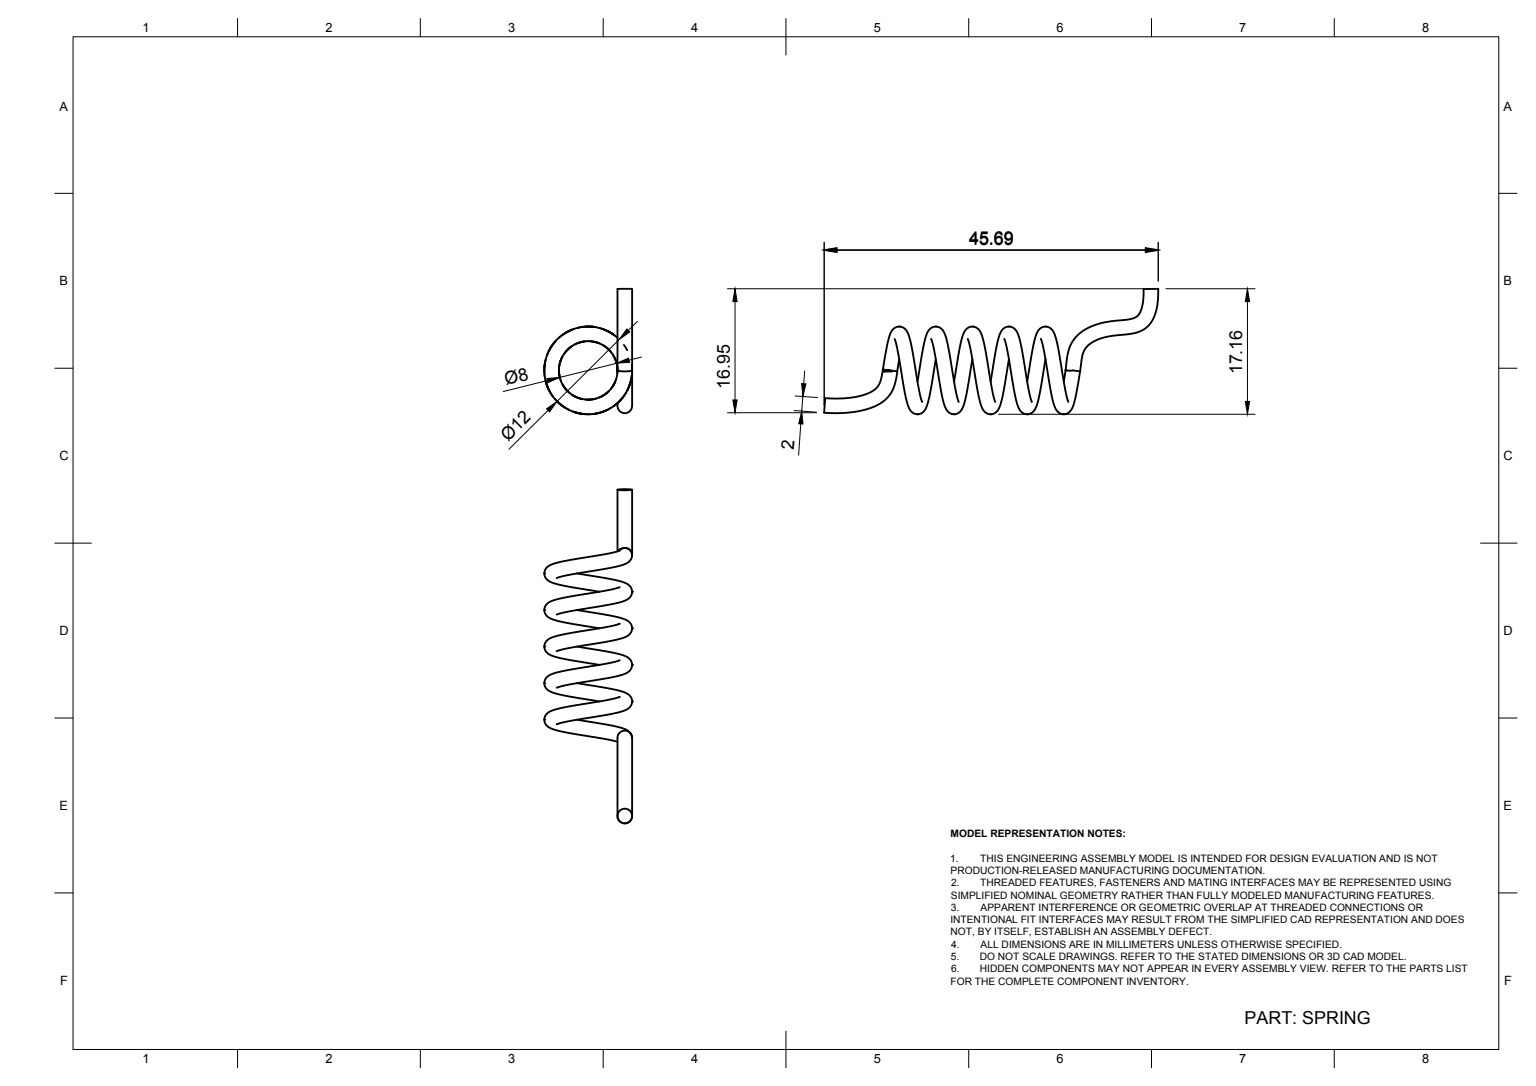
ISO-10303-21;
HEADER;
/* Generated by software containing ST-Developer
 * from STEP Tools, Inc. (www.steptools.com) 
 */

FILE_DESCRIPTION(
/* description */ (''),
/* implementation_level */ '2;1');

FILE_NAME(
/* name */ 'Spring.step',
/* time_stamp */ '2026-09-20T22:38:01+06:00',
/* author */ (''),
/* organization */ (''),
/* preprocessor_version */ 'ST-DEVELOPER v20.2',
/* originating_system */ 'Autodesk Translation Framework v15.15.0.0',
/* authorisation */ '');

FILE_SCHEMA (('AUTOMOTIVE_DESIGN { 1 0 10303 214 3 1 1 }'));
ENDSEC;

DATA;
#10=MECHANICAL_DESIGN_GEOMETRIC_PRESENTATION_REPRESENTATION('',(#86),#4079);
#43=B_SPLINE_CURVE_WITH_KNOTS('',3,(#2659,#2660,#2661,#2662,#2663,#2664,
#2665,#2666,#2667,#2668,#2669,#2670,#2671,#2672,#2673,#2674,#2675,#2676,
#2677,#2678,#2679,#2680,#2681,#2682,#2683,#2684,#2685,#2686),
 .UNSPECIFIED.,.F.,.F.,(4,3,3,3,3,3,3,3,3,4),(-0.465553767595507,-0.45230342916427,
-0.438736142747031,-0.431079433868877,-0.417558478811202,-0.404199900672923,
-0.391686604552913,-0.378322214394046,-0.374830772248012,-0.369773118077988),
 .UNSPECIFIED.);
#44=B_SPLINE_CURVE_WITH_KNOTS('',3,(#2688,#2689,#2690,#2691,#2692,#2693,
#2694,#2695,#2696,#2697),.UNSPECIFIED.,.F.,.F.,(4,2,2,2,4),(-0.09742200167385,
-0.0775242929113368,-0.0386624365460309,0.,0.00241811618144354),
 .UNSPECIFIED.);
#45=B_SPLINE_CURVE_WITH_KNOTS('',3,(#2702,#2703,#2704,#2705,#2706,#2707,
#2708,#2709,#2710,#2711),.UNSPECIFIED.,.F.,.F.,(4,3,3,4),(-0.657219142658169,
-0.648664678619421,-0.598426048115365,-0.569492481999336),.UNSPECIFIED.);
#46=B_SPLINE_CURVE_WITH_KNOTS('',3,(#2712,#2713,#2714,#2715,#2716,#2717,
#2718,#2719,#2720,#2721),.UNSPECIFIED.,.F.,.F.,(4,3,3,4),(-0.489269526390867,
-0.47602824474659,-0.470821216724862,-0.465553767595507),.UNSPECIFIED.);
#47=B_SPLINE_CURVE_WITH_KNOTS('',3,(#2723,#2724,#2725,#2726,#2727,#2728,
#2729,#2730,#2731),.UNSPECIFIED.,.F.,.F.,(4,1,1,1,1,1,4),(0.0132171477861262,
0.142857142857143,0.285714285714286,0.428571428571429,0.571428571428571,
0.857142857142857,1.),.UNSPECIFIED.);
#48=B_SPLINE_CURVE_WITH_KNOTS('',3,(#3403,#3404,#3405,#3406,#3407,#3408,
#3409,#3410,#3411,#3412,#3413,#3414,#3415,#3416,#3417,#3418,#3419,#3420,
#3421,#3422,#3423,#3424,#3425),.UNSPECIFIED.,.F.,.F.,(4,2,3,2,2,2,2,2,2,
2,4),(0.587267836178956,0.604560146171109,0.626248329271999,0.664698946888708,
0.70347541138122,0.74264809527987,0.78210152700143,0.821492769940296,0.860375715352057,
0.898588405045022,0.900352617840992),.UNSPECIFIED.);
#49=B_SPLINE_CURVE_WITH_KNOTS('',3,(#3427,#3428,#3429,#3430,#3431,#3432,
#3433,#3434,#3435,#3436,#3437,#3438,#3439,#3440,#3441,#3442,#3443,#3444,
#3445,#3446,#3447,#3448,#3449,#3450,#3451,#3452,#3453,#3454,#3455,#3456,
#3457,#3458,#3459,#3460,#3461,#3462,#3463,#3464,#3465,#3466,#3467,#3468,
#3469,#3470,#3471,#3472,#3473,#3474,#3475,#3476,#3477,#3478,#3479,#3480,
#3481,#3482,#3483,#3484,#3485,#3486,#3487,#3488,#3489,#3490,#3491,#3492,
#3493),.UNSPECIFIED.,.F.,.F.,(4,1,1,1,1,1,1,1,1,1,1,1,1,1,1,1,1,1,1,1,1,
1,1,1,1,1,1,1,1,1,1,1,1,1,1,1,1,1,1,1,1,1,1,1,1,1,1,1,1,1,1,1,1,1,1,1,1,
1,1,1,1,1,1,1,4),(0.,0.464577110944849,0.95586837165839,1.44715963237193,
1.93845089308547,2.42974215379901,2.92103341451255,3.41232467522609,3.90361593593964,
4.39490719665318,4.88619845736672,5.37748971808026,5.8687809787938,6.36007223950734,
6.85136350022088,7.34265476093442,7.83394602164796,8.3252372823615,8.81652854307505,
9.30781980378859,9.79911106450213,10.2904023252157,10.7816935859292,11.2729848466427,
11.7642761073563,12.2555673680698,12.7468586287834,13.2381498894969,13.7294411502105,
14.220732410924,14.7120236716375,15.2033149323511,15.6946061930646,16.1858974537782,
16.6771887144917,17.1684799752052,17.6597712359188,18.1510624966323,18.6423537573459,
19.1336450180594,19.6249362787729,20.1162275394865,20.6075188002,21.0988100609136,
21.5901013216271,22.0813925823407,22.5726838430542,23.0639751037677,23.5552663644813,
24.0465576251948,24.5378488859084,25.0291401466219,25.5204314073354,26.011722668049,
26.5030139287625,26.9943051894761,27.4855964501896,27.9768877109031,28.4681789716167,
28.9594702323302,29.4507614930438,29.9420527537573,30.4333440144708,30.9246352751844,
31.4159265358979),.UNSPECIFIED.);
#50=B_SPLINE_CURVE_WITH_KNOTS('',3,(#3495,#3496,#3497,#3498,#3499,#3500,
#3501,#3502,#3503,#3504,#3505,#3506,#3507,#3508,#3509,#3510,#3511,#3512,
#3513,#3514),.UNSPECIFIED.,.F.,.F.,(4,2,2,2,2,2,2,2,2,4),(-0.313052705156199,
-0.292609441796844,-0.272153993775093,-0.233472325120928,-0.194370984993977,
-0.154905297587714,-0.115391052867927,-0.0763129985395409,-0.0379453287021336,
0.),.UNSPECIFIED.);
#51=B_SPLINE_CURVE_WITH_KNOTS('',3,(#3516,#3517,#3518,#3519,#3520,#3521,
#3522,#3523,#3524,#3525,#3526,#3527,#3528,#3529,#3530,#3531),
 .UNSPECIFIED.,.F.,.F.,(4,3,3,3,3,4),(-0.0024248849541149,0.,0.0138283319525736,
0.0273768962823761,0.0362935842092716,0.0434201122759664),.UNSPECIFIED.);
#52=B_SPLINE_CURVE_WITH_KNOTS('',3,(#3533,#3534,#3535,#3536,#3537,#3538),
 .UNSPECIFIED.,.F.,.F.,(4,2,4),(-0.0515505060017679,-0.0391387739403107,
0.),.UNSPECIFIED.);
#53=B_SPLINE_CURVE_WITH_KNOTS('',3,(#3542,#3543,#3544,#3545,#3546,#3547,
#3548,#3549,#3550,#3551,#3552,#3553,#3554,#3555,#3556,#3557,#3558,#3559,
#3560,#3561),.UNSPECIFIED.,.F.,.F.,(4,2,2,2,2,2,2,2,2,4),(-0.313052705156207,
-0.29260944179685,-0.272153993775096,-0.233472325120924,-0.194370984993967,
-0.154905297587702,-0.11539105286792,-0.0763129985395404,-0.0379453287021338,
0.),.UNSPECIFIED.);
#54=B_SPLINE_CURVE_WITH_KNOTS('',3,(#3563,#3564,#3565,#3566,#3567,#3568,
#3569,#3570,#3571,#3572,#3573,#3574,#3575,#3576,#3577,#3578,#3579,#3580,
#3581,#3582,#3583,#3584,#3585,#3586,#3587,#3588,#3589,#3590,#3591,#3592,
#3593,#3594,#3595,#3596),.UNSPECIFIED.,.F.,.F.,(4,3,3,3,3,3,3,3,3,3,3,4),
(0.377352254196932,0.390588465654341,0.403867575958707,0.41718187397498,
0.429352359462404,0.437218808334642,0.450427222970435,0.463782588613302,
0.468146972739535,0.481501401691605,0.494833441685106,0.497267224677679),
 .UNSPECIFIED.);
#55=B_SPLINE_CURVE_WITH_KNOTS('',3,(#3600,#3601,#3602,#3603,#3604,#3605,
#3606,#3607,#3608,#3609,#3610,#3611,#3612,#3613,#3614,#3615,#3616,#3617,
#3618,#3619,#3620,#3621,#3622,#3623,#3624,#3625,#3626,#3627),
 .UNSPECIFIED.,.F.,.F.,(4,3,3,3,3,3,3,3,3,4),(0.458621120799817,0.464048968999107,
0.469643578756217,0.482746851650584,0.496256676637028,0.508878670584022,
0.522421915099756,0.535791652499991,0.548459753273671,0.554671659389392),
 .UNSPECIFIED.);
#56=B_SPLINE_CURVE_WITH_KNOTS('',3,(#3888,#3889,#3890,#3891,#3892,#3893,
#3894,#3895,#3896,#3897),.UNSPECIFIED.,.F.,.F.,(4,3,3,4),(-0.319964114535563,
-0.319531325306217,-0.229500308639694,-0.144878157103041),.UNSPECIFIED.);
#57=B_SPLINE_CURVE_WITH_KNOTS('',3,(#3900,#3901,#3902,#3903,#3904,#3905,
#3906,#3907,#3908,#3909,#3910,#3911,#3912,#3913,#3914,#3915,#3916,#3917,
#3918,#3919,#3920,#3921,#3922,#3923),.UNSPECIFIED.,.F.,.F.,(4,1,1,1,1,1,
1,1,1,1,1,1,1,1,1,1,1,1,1,1,1,4),(0.,0.025,0.05,0.1,0.15,0.175,0.2,0.3,
0.4,0.425,0.45,0.5,0.55,0.575,0.6,0.7,0.75,0.8,0.825,0.85,0.9,1.),
 .UNSPECIFIED.);
#58=B_SPLINE_SURFACE_WITH_KNOTS('',3,3,((#2567,#2568,#2569,#2570,#2571,
#2572,#2573,#2574,#2575),(#2576,#2577,#2578,#2579,#2580,#2581,#2582,#2583,
#2584),(#2585,#2586,#2587,#2588,#2589,#2590,#2591,#2592,#2593),(#2594,#2595,
#2596,#2597,#2598,#2599,#2600,#2601,#2602),(#2603,#2604,#2605,#2606,#2607,
#2608,#2609,#2610,#2611),(#2612,#2613,#2614,#2615,#2616,#2617,#2618,#2619,
#2620),(#2621,#2622,#2623,#2624,#2625,#2626,#2627,#2628,#2629),(#2630,#2631,
#2632,#2633,#2634,#2635,#2636,#2637,#2638),(#2639,#2640,#2641,#2642,#2643,
#2644,#2645,#2646,#2647),(#2648,#2649,#2650,#2651,#2652,#2653,#2654,#2655,
#2656)),.UNSPECIFIED.,.T.,.F.,.F.,(4,1,1,1,1,1,1,4),(4,1,1,1,1,1,4),(-3.14159265359034,
-2.2439947525646,-1.34639685153886,-0.448798950513122,0.448798950512615,
1.34639685153835,2.24399475256409,3.14159265358983),(0.,0.142857142857143,
0.285714285714286,0.428571428571429,0.571428571428571,0.857142857142857,
1.),.UNSPECIFIED.);
#59=B_SPLINE_SURFACE_WITH_KNOTS('',3,3,((#2733,#2734,#2735,#2736,#2737,
#2738,#2739,#2740,#2741,#2742,#2743,#2744,#2745,#2746,#2747,#2748,#2749,
#2750,#2751,#2752,#2753,#2754,#2755,#2756,#2757,#2758,#2759,#2760,#2761,
#2762,#2763,#2764,#2765,#2766,#2767,#2768,#2769,#2770,#2771,#2772,#2773,
#2774,#2775,#2776,#2777,#2778,#2779,#2780,#2781,#2782,#2783,#2784,#2785,
#2786,#2787,#2788,#2789,#2790,#2791,#2792,#2793,#2794,#2795,#2796,#2797,
#2798,#2799),(#2800,#2801,#2802,#2803,#2804,#2805,#2806,#2807,#2808,#2809,
#2810,#2811,#2812,#2813,#2814,#2815,#2816,#2817,#2818,#2819,#2820,#2821,
#2822,#2823,#2824,#2825,#2826,#2827,#2828,#2829,#2830,#2831,#2832,#2833,
#2834,#2835,#2836,#2837,#2838,#2839,#2840,#2841,#2842,#2843,#2844,#2845,
#2846,#2847,#2848,#2849,#2850,#2851,#2852,#2853,#2854,#2855,#2856,#2857,
#2858,#2859,#2860,#2861,#2862,#2863,#2864,#2865,#2866),(#2867,#2868,#2869,
#2870,#2871,#2872,#2873,#2874,#2875,#2876,#2877,#2878,#2879,#2880,#2881,
#2882,#2883,#2884,#2885,#2886,#2887,#2888,#2889,#2890,#2891,#2892,#2893,
#2894,#2895,#2896,#2897,#2898,#2899,#2900,#2901,#2902,#2903,#2904,#2905,
#2906,#2907,#2908,#2909,#2910,#2911,#2912,#2913,#2914,#2915,#2916,#2917,
#2918,#2919,#2920,#2921,#2922,#2923,#2924,#2925,#2926,#2927,#2928,#2929,
#2930,#2931,#2932,#2933),(#2934,#2935,#2936,#2937,#2938,#2939,#2940,#2941,
#2942,#2943,#2944,#2945,#2946,#2947,#2948,#2949,#2950,#2951,#2952,#2953,
#2954,#2955,#2956,#2957,#2958,#2959,#2960,#2961,#2962,#2963,#2964,#2965,
#2966,#2967,#2968,#2969,#2970,#2971,#2972,#2973,#2974,#2975,#2976,#2977,
#2978,#2979,#2980,#2981,#2982,#2983,#2984,#2985,#2986,#2987,#2988,#2989,
#2990,#2991,#2992,#2993,#2994,#2995,#2996,#2997,#2998,#2999,#3000),(#3001,
#3002,#3003,#3004,#3005,#3006,#3007,#3008,#3009,#3010,#3011,#3012,#3013,
#3014,#3015,#3016,#3017,#3018,#3019,#3020,#3021,#3022,#3023,#3024,#3025,
#3026,#3027,#3028,#3029,#3030,#3031,#3032,#3033,#3034,#3035,#3036,#3037,
#3038,#3039,#3040,#3041,#3042,#3043,#3044,#3045,#3046,#3047,#3048,#3049,
#3050,#3051,#3052,#3053,#3054,#3055,#3056,#3057,#3058,#3059,#3060,#3061,
#3062,#3063,#3064,#3065,#3066,#3067),(#3068,#3069,#3070,#3071,#3072,#3073,
#3074,#3075,#3076,#3077,#3078,#3079,#3080,#3081,#3082,#3083,#3084,#3085,
#3086,#3087,#3088,#3089,#3090,#3091,#3092,#3093,#3094,#3095,#3096,#3097,
#3098,#3099,#3100,#3101,#3102,#3103,#3104,#3105,#3106,#3107,#3108,#3109,
#3110,#3111,#3112,#3113,#3114,#3115,#3116,#3117,#3118,#3119,#3120,#3121,
#3122,#3123,#3124,#3125,#3126,#3127,#3128,#3129,#3130,#3131,#3132,#3133,
#3134),(#3135,#3136,#3137,#3138,#3139,#3140,#3141,#3142,#3143,#3144,#3145,
#3146,#3147,#3148,#3149,#3150,#3151,#3152,#3153,#3154,#3155,#3156,#3157,
#3158,#3159,#3160,#3161,#3162,#3163,#3164,#3165,#3166,#3167,#3168,#3169,
#3170,#3171,#3172,#3173,#3174,#3175,#3176,#3177,#3178,#3179,#3180,#3181,
#3182,#3183,#3184,#3185,#3186,#3187,#3188,#3189,#3190,#3191,#3192,#3193,
#3194,#3195,#3196,#3197,#3198,#3199,#3200,#3201),(#3202,#3203,#3204,#3205,
#3206,#3207,#3208,#3209,#3210,#3211,#3212,#3213,#3214,#3215,#3216,#3217,
#3218,#3219,#3220,#3221,#3222,#3223,#3224,#3225,#3226,#3227,#3228,#3229,
#3230,#3231,#3232,#3233,#3234,#3235,#3236,#3237,#3238,#3239,#3240,#3241,
#3242,#3243,#3244,#3245,#3246,#3247,#3248,#3249,#3250,#3251,#3252,#3253,
#3254,#3255,#3256,#3257,#3258,#3259,#3260,#3261,#3262,#3263,#3264,#3265,
#3266,#3267,#3268),(#3269,#3270,#3271,#3272,#3273,#3274,#3275,#3276,#3277,
#3278,#3279,#3280,#3281,#3282,#3283,#3284,#3285,#3286,#3287,#3288,#3289,
#3290,#3291,#3292,#3293,#3294,#3295,#3296,#3297,#3298,#3299,#3300,#3301,
#3302,#3303,#3304,#3305,#3306,#3307,#3308,#3309,#3310,#3311,#3312,#3313,
#3314,#3315,#3316,#3317,#3318,#3319,#3320,#3321,#3322,#3323,#3324,#3325,
#3326,#3327,#3328,#3329,#3330,#3331,#3332,#3333,#3334,#3335),(#3336,#3337,
#3338,#3339,#3340,#3341,#3342,#3343,#3344,#3345,#3346,#3347,#3348,#3349,
#3350,#3351,#3352,#3353,#3354,#3355,#3356,#3357,#3358,#3359,#3360,#3361,
#3362,#3363,#3364,#3365,#3366,#3367,#3368,#3369,#3370,#3371,#3372,#3373,
#3374,#3375,#3376,#3377,#3378,#3379,#3380,#3381,#3382,#3383,#3384,#3385,
#3386,#3387,#3388,#3389,#3390,#3391,#3392,#3393,#3394,#3395,#3396,#3397,
#3398,#3399,#3400,#3401,#3402)),.UNSPECIFIED.,.T.,.F.,.F.,(4,1,1,1,1,1,
1,4),(4,1,1,1,1,1,1,1,1,1,1,1,1,1,1,1,1,1,1,1,1,1,1,1,1,1,1,1,1,1,1,1,1,
1,1,1,1,1,1,1,1,1,1,1,1,1,1,1,1,1,1,1,1,1,1,1,1,1,1,1,1,1,1,1,4),(-3.14159265358979,
-2.24399475256414,-1.34639685153848,-0.448798950512828,0.448798950512828,
1.34639685153848,2.24399475256414,3.14159265358979),(-0.0267141497686917,
0.464577110944849,0.95586837165839,1.44715963237193,1.93845089308547,2.42974215379901,
2.92103341451255,3.41232467522609,3.90361593593964,4.39490719665318,4.88619845736672,
5.37748971808026,5.8687809787938,6.36007223950734,6.85136350022088,7.34265476093442,
7.83394602164796,8.3252372823615,8.81652854307505,9.30781980378859,9.79911106450213,
10.2904023252157,10.7816935859292,11.2729848466427,11.7642761073563,12.2555673680698,
12.7468586287834,13.2381498894969,13.7294411502105,14.220732410924,14.7120236716375,
15.2033149323511,15.6946061930646,16.1858974537782,16.6771887144917,17.1684799752052,
17.6597712359188,18.1510624966323,18.6423537573459,19.1336450180594,19.6249362787729,
20.1162275394865,20.6075188002,21.0988100609136,21.5901013216271,22.0813925823407,
22.5726838430542,23.0639751037677,23.5552663644813,24.0465576251948,24.5378488859084,
25.0291401466219,25.5204314073354,26.011722668049,26.5030139287625,26.9943051894761,
27.4855964501896,27.9768877109031,28.4681789716167,28.9594702323302,29.4507614930438,
29.9420527537573,30.4333440144708,30.9246352751844,31.4159265358979),
 .UNSPECIFIED.);
#60=B_SPLINE_SURFACE_WITH_KNOTS('',3,3,((#3628,#3629,#3630,#3631,#3632,
#3633,#3634,#3635,#3636,#3637,#3638,#3639,#3640,#3641,#3642,#3643,#3644,
#3645,#3646,#3647,#3648,#3649,#3650,#3651,#3652,#3653),(#3654,#3655,#3656,
#3657,#3658,#3659,#3660,#3661,#3662,#3663,#3664,#3665,#3666,#3667,#3668,
#3669,#3670,#3671,#3672,#3673,#3674,#3675,#3676,#3677,#3678,#3679),(#3680,
#3681,#3682,#3683,#3684,#3685,#3686,#3687,#3688,#3689,#3690,#3691,#3692,
#3693,#3694,#3695,#3696,#3697,#3698,#3699,#3700,#3701,#3702,#3703,#3704,
#3705),(#3706,#3707,#3708,#3709,#3710,#3711,#3712,#3713,#3714,#3715,#3716,
#3717,#3718,#3719,#3720,#3721,#3722,#3723,#3724,#3725,#3726,#3727,#3728,
#3729,#3730,#3731),(#3732,#3733,#3734,#3735,#3736,#3737,#3738,#3739,#3740,
#3741,#3742,#3743,#3744,#3745,#3746,#3747,#3748,#3749,#3750,#3751,#3752,
#3753,#3754,#3755,#3756,#3757),(#3758,#3759,#3760,#3761,#3762,#3763,#3764,
#3765,#3766,#3767,#3768,#3769,#3770,#3771,#3772,#3773,#3774,#3775,#3776,
#3777,#3778,#3779,#3780,#3781,#3782,#3783),(#3784,#3785,#3786,#3787,#3788,
#3789,#3790,#3791,#3792,#3793,#3794,#3795,#3796,#3797,#3798,#3799,#3800,
#3801,#3802,#3803,#3804,#3805,#3806,#3807,#3808,#3809),(#3810,#3811,#3812,
#3813,#3814,#3815,#3816,#3817,#3818,#3819,#3820,#3821,#3822,#3823,#3824,
#3825,#3826,#3827,#3828,#3829,#3830,#3831,#3832,#3833,#3834,#3835),(#3836,
#3837,#3838,#3839,#3840,#3841,#3842,#3843,#3844,#3845,#3846,#3847,#3848,
#3849,#3850,#3851,#3852,#3853,#3854,#3855,#3856,#3857,#3858,#3859,#3860,
#3861),(#3862,#3863,#3864,#3865,#3866,#3867,#3868,#3869,#3870,#3871,#3872,
#3873,#3874,#3875,#3876,#3877,#3878,#3879,#3880,#3881,#3882,#3883,#3884,
#3885,#3886,#3887)),.UNSPECIFIED.,.T.,.F.,.F.,(4,1,1,1,1,1,1,4),(4,2,1,
1,1,1,1,1,1,1,1,1,1,1,1,1,1,1,1,1,1,1,4),(-3.14159265358979,-2.24399475256414,
-1.34639685153848,-0.448798950512828,0.448798950512828,1.34639685153848,
2.24399475256414,3.14159265358979),(-0.00680747846147418,0.,0.025,0.05,
0.1,0.15,0.175,0.2,0.3,0.4,0.425,0.45,0.5,0.55,0.575,0.6,0.7,0.75,0.8,0.825,
0.85,0.9,1.),.UNSPECIFIED.);
#61=B_SPLINE_SURFACE_WITH_KNOTS('',3,3,((#3925,#3926,#3927,#3928),(#3929,
#3930,#3931,#3932),(#3933,#3934,#3935,#3936),(#3937,#3938,#3939,#3940),
(#3941,#3942,#3943,#3944)),.UNSPECIFIED.,.F.,.F.,.F.,(4,1,4),(4,4),(-0.950877784735382,
-0.352362581588169,0.246152621559044),(-0.0375396701634702,0.),
 .UNSPECIFIED.);
#70=SHAPE_REPRESENTATION_RELATIONSHIP('SRR','None',#4113,#78);
#78=ADVANCED_BREP_SHAPE_REPRESENTATION('',(#94),#4073);
#86=STYLED_ITEM('',(#4162),#94);
#94=MANIFOLD_SOLID_BREP('Spring',#1445);
#150=CIRCLE('',#1633,1.);
#151=CIRCLE('',#1634,1.);
#152=CIRCLE('',#1635,1.);
#153=CIRCLE('',#1636,1.);
#154=CIRCLE('',#1637,1.);
#155=CIRCLE('',#1640,1.);
#156=CIRCLE('',#1641,1.);
#244=FACE_OUTER_BOUND('',#332,.T.);
#245=FACE_OUTER_BOUND('',#333,.T.);
#246=FACE_OUTER_BOUND('',#334,.T.);
#247=FACE_OUTER_BOUND('',#335,.T.);
#248=FACE_OUTER_BOUND('',#336,.T.);
#249=FACE_OUTER_BOUND('',#337,.T.);
#250=FACE_OUTER_BOUND('',#338,.T.);
#251=FACE_OUTER_BOUND('',#339,.T.);
#252=FACE_OUTER_BOUND('',#340,.T.);
#253=FACE_OUTER_BOUND('',#341,.T.);
#254=FACE_OUTER_BOUND('',#342,.T.);
#255=FACE_OUTER_BOUND('',#343,.T.);
#256=FACE_OUTER_BOUND('',#344,.T.);
#332=EDGE_LOOP('',(#1177,#1178,#1179,#1180,#1181,#1182,#1183,#1184,#1185));
#333=EDGE_LOOP('',(#1186,#1187,#1188,#1189,#1190,#1191,#1192,#1193,#1194));
#334=EDGE_LOOP('',(#1195,#1196,#1197));
#335=EDGE_LOOP('',(#1198,#1199,#1200));
#336=EDGE_LOOP('',(#1201,#1202,#1203,#1204,#1205,#1206,#1207));
#337=EDGE_LOOP('',(#1208,#1209,#1210));
#338=EDGE_LOOP('',(#1211,#1212));
#339=EDGE_LOOP('',(#1213,#1214));
#340=EDGE_LOOP('',(#1215));
#341=EDGE_LOOP('',(#1216,#1217,#1218,#1219));
#342=EDGE_LOOP('',(#1220,#1221));
#343=EDGE_LOOP('',(#1222));
#344=EDGE_LOOP('',(#1223,#1224));
#452=LINE('',#3599,#565);
#453=LINE('',#3949,#566);
#565=VECTOR('',#1979,10.);
#566=VECTOR('',#1992,10.);
#683=VERTEX_POINT('',#2657);
#684=VERTEX_POINT('',#2658);
#685=VERTEX_POINT('',#2687);
#686=VERTEX_POINT('',#2698);
#687=VERTEX_POINT('',#2701);
#688=VERTEX_POINT('',#2722);
#689=VERTEX_POINT('',#3426);
#690=VERTEX_POINT('',#3494);
#691=VERTEX_POINT('',#3515);
#692=VERTEX_POINT('',#3532);
#693=VERTEX_POINT('',#3539);
#694=VERTEX_POINT('',#3598);
#695=VERTEX_POINT('',#3899);
#853=EDGE_CURVE('',#683,#684,#43,.T.);
#854=EDGE_CURVE('',#684,#685,#44,.T.);
#855=EDGE_CURVE('',#685,#686,#150,.T.);
#856=EDGE_CURVE('',#686,#685,#151,.T.);
#857=EDGE_CURVE('',#685,#687,#45,.T.);
#858=EDGE_CURVE('',#687,#683,#46,.T.);
#859=EDGE_CURVE('',#683,#688,#47,.T.);
#860=EDGE_CURVE('',#688,#688,#152,.T.);
#861=EDGE_CURVE('',#686,#685,#48,.T.);
#862=EDGE_CURVE('',#686,#689,#49,.T.);
#863=EDGE_CURVE('',#689,#690,#50,.T.);
#864=EDGE_CURVE('',#690,#691,#51,.T.);
#865=EDGE_CURVE('',#691,#692,#52,.T.);
#866=EDGE_CURVE('',#693,#692,#153,.T.);
#867=EDGE_CURVE('',#693,#689,#154,.T.);
#868=EDGE_CURVE('',#686,#685,#53,.T.);
#869=EDGE_CURVE('',#684,#687,#54,.T.);
#870=EDGE_CURVE('',#693,#694,#452,.T.);
#871=EDGE_CURVE('',#694,#689,#55,.T.);
#872=EDGE_CURVE('',#691,#694,#56,.T.);
#873=EDGE_CURVE('',#690,#689,#155,.T.);
#874=EDGE_CURVE('',#689,#695,#57,.T.);
#875=EDGE_CURVE('',#695,#695,#156,.T.);
#876=EDGE_CURVE('',#692,#693,#453,.F.);
#1177=ORIENTED_EDGE('',*,*,#853,.T.);
#1178=ORIENTED_EDGE('',*,*,#854,.T.);
#1179=ORIENTED_EDGE('',*,*,#855,.T.);
#1180=ORIENTED_EDGE('',*,*,#856,.T.);
#1181=ORIENTED_EDGE('',*,*,#857,.T.);
#1182=ORIENTED_EDGE('',*,*,#858,.T.);
#1183=ORIENTED_EDGE('',*,*,#859,.T.);
#1184=ORIENTED_EDGE('',*,*,#860,.F.);
#1185=ORIENTED_EDGE('',*,*,#859,.F.);
#1186=ORIENTED_EDGE('',*,*,#861,.F.);
#1187=ORIENTED_EDGE('',*,*,#862,.T.);
#1188=ORIENTED_EDGE('',*,*,#863,.T.);
#1189=ORIENTED_EDGE('',*,*,#864,.T.);
#1190=ORIENTED_EDGE('',*,*,#865,.T.);
#1191=ORIENTED_EDGE('',*,*,#866,.F.);
#1192=ORIENTED_EDGE('',*,*,#867,.T.);
#1193=ORIENTED_EDGE('',*,*,#862,.F.);
#1194=ORIENTED_EDGE('',*,*,#868,.T.);
#1195=ORIENTED_EDGE('',*,*,#858,.F.);
#1196=ORIENTED_EDGE('',*,*,#869,.F.);
#1197=ORIENTED_EDGE('',*,*,#853,.F.);
#1198=ORIENTED_EDGE('',*,*,#867,.F.);
#1199=ORIENTED_EDGE('',*,*,#870,.T.);
#1200=ORIENTED_EDGE('',*,*,#871,.T.);
#1201=ORIENTED_EDGE('',*,*,#872,.F.);
#1202=ORIENTED_EDGE('',*,*,#864,.F.);
#1203=ORIENTED_EDGE('',*,*,#873,.T.);
#1204=ORIENTED_EDGE('',*,*,#874,.T.);
#1205=ORIENTED_EDGE('',*,*,#875,.F.);
#1206=ORIENTED_EDGE('',*,*,#874,.F.);
#1207=ORIENTED_EDGE('',*,*,#871,.F.);
#1208=ORIENTED_EDGE('',*,*,#854,.F.);
#1209=ORIENTED_EDGE('',*,*,#869,.T.);
#1210=ORIENTED_EDGE('',*,*,#857,.F.);
#1211=ORIENTED_EDGE('',*,*,#855,.F.);
#1212=ORIENTED_EDGE('',*,*,#868,.F.);
#1213=ORIENTED_EDGE('',*,*,#861,.T.);
#1214=ORIENTED_EDGE('',*,*,#856,.F.);
#1215=ORIENTED_EDGE('',*,*,#860,.T.);
#1216=ORIENTED_EDGE('',*,*,#865,.F.);
#1217=ORIENTED_EDGE('',*,*,#872,.T.);
#1218=ORIENTED_EDGE('',*,*,#870,.F.);
#1219=ORIENTED_EDGE('',*,*,#876,.F.);
#1220=ORIENTED_EDGE('',*,*,#863,.F.);
#1221=ORIENTED_EDGE('',*,*,#873,.F.);
#1222=ORIENTED_EDGE('',*,*,#875,.T.);
#1223=ORIENTED_EDGE('',*,*,#876,.T.);
#1224=ORIENTED_EDGE('',*,*,#866,.T.);
#1332=PLANE('',#1638);
#1333=PLANE('',#1639);
#1334=PLANE('',#1642);
#1335=PLANE('',#1643);
#1336=PLANE('',#1644);
#1337=PLANE('',#1645);
#1338=PLANE('',#1646);
#1339=PLANE('',#1647);
#1340=PLANE('',#1648);
#1406=ADVANCED_FACE('',(#244),#58,.T.);
#1407=ADVANCED_FACE('',(#245),#59,.T.);
#1408=ADVANCED_FACE('',(#246),#1332,.F.);
#1409=ADVANCED_FACE('',(#247),#1333,.F.);
#1410=ADVANCED_FACE('',(#248),#60,.T.);
#1411=ADVANCED_FACE('',(#249),#61,.T.);
#1412=ADVANCED_FACE('',(#250),#1334,.F.);
#1413=ADVANCED_FACE('',(#251),#1335,.F.);
#1414=ADVANCED_FACE('',(#252),#1336,.T.);
#1415=ADVANCED_FACE('',(#253),#1337,.F.);
#1416=ADVANCED_FACE('',(#254),#1338,.F.);
#1417=ADVANCED_FACE('',(#255),#1339,.T.);
#1418=ADVANCED_FACE('',(#256),#1340,.T.);
#1445=CLOSED_SHELL('',(#1406,#1407,#1408,#1409,#1410,#1411,#1412,#1413,
#1414,#1415,#1416,#1417,#1418));
#1632=AXIS2_PLACEMENT_3D('',#2566,#1963,#1964);
#1633=AXIS2_PLACEMENT_3D('',#2699,#1965,#1966);
#1634=AXIS2_PLACEMENT_3D('',#2700,#1967,#1968);
#1635=AXIS2_PLACEMENT_3D('',#2732,#1969,#1970);
#1636=AXIS2_PLACEMENT_3D('',#3540,#1971,#1972);
#1637=AXIS2_PLACEMENT_3D('',#3541,#1973,#1974);
#1638=AXIS2_PLACEMENT_3D('',#3562,#1975,#1976);
#1639=AXIS2_PLACEMENT_3D('',#3597,#1977,#1978);
#1640=AXIS2_PLACEMENT_3D('',#3898,#1980,#1981);
#1641=AXIS2_PLACEMENT_3D('',#3924,#1982,#1983);
#1642=AXIS2_PLACEMENT_3D('',#3945,#1984,#1985);
#1643=AXIS2_PLACEMENT_3D('',#3946,#1986,#1987);
#1644=AXIS2_PLACEMENT_3D('',#3947,#1988,#1989);
#1645=AXIS2_PLACEMENT_3D('',#3948,#1990,#1991);
#1646=AXIS2_PLACEMENT_3D('',#3950,#1993,#1994);
#1647=AXIS2_PLACEMENT_3D('',#3951,#1995,#1996);
#1648=AXIS2_PLACEMENT_3D('',#3952,#1997,#1998);
#1963=DIRECTION('axis',(0.,0.,1.));
#1964=DIRECTION('refdir',(1.,0.,0.));
#1965=DIRECTION('center_axis',(0.,-0.991319117631768,-0.131477781460493));
#1966=DIRECTION('ref_axis',(1.,0.,0.));
#1967=DIRECTION('center_axis',(0.,-0.991319117631768,-0.131477781460493));
#1968=DIRECTION('ref_axis',(1.,0.,0.));
#1969=DIRECTION('center_axis',(0.,0.072334353589932,-0.997380439597011));
#1970=DIRECTION('ref_axis',(1.,0.,0.));
#1971=DIRECTION('center_axis',(1.22464679914735E-15,1.,0.));
#1972=DIRECTION('ref_axis',(-1.,1.22464679914735E-15,0.));
#1973=DIRECTION('center_axis',(-1.22464679914735E-15,-1.,0.));
#1974=DIRECTION('ref_axis',(-1.,1.22464679914735E-15,0.));
#1975=DIRECTION('center_axis',(0.,1.,0.));
#1976=DIRECTION('ref_axis',(0.,0.,1.));
#1977=DIRECTION('center_axis',(1.22464679914735E-15,1.,0.));
#1978=DIRECTION('ref_axis',(0.,0.,1.));
#1979=DIRECTION('',(1.,-1.22464679914735E-15,9.23361932986486E-15));
#1980=DIRECTION('center_axis',(0.,0.991319117631768,0.13147778146049));
#1981=DIRECTION('ref_axis',(-1.,0.,0.));
#1982=DIRECTION('center_axis',(0.,0.999879786123581,-0.0155052668942604));
#1983=DIRECTION('ref_axis',(-1.,0.,0.));
#1984=DIRECTION('center_axis',(0.,-0.991319117631768,-0.131477781460493));
#1985=DIRECTION('ref_axis',(0.,0.131477781460493,-0.991319117631768));
#1986=DIRECTION('center_axis',(0.,-0.991319117631768,-0.131477781460493));
#1987=DIRECTION('ref_axis',(0.,0.131477781460493,-0.991319117631768));
#1988=DIRECTION('center_axis',(0.,0.072334353589932,-0.997380439597011));
#1989=DIRECTION('ref_axis',(0.,0.997380439597011,0.072334353589932));
#1990=DIRECTION('center_axis',(0.,0.991319117631768,0.13147778146049));
#1991=DIRECTION('ref_axis',(0.,-0.13147778146049,0.991319117631768));
#1992=DIRECTION('',(-1.,1.22464679914735E-15,-9.23361932986486E-15));
#1993=DIRECTION('center_axis',(0.,0.991319117631768,0.13147778146049));
#1994=DIRECTION('ref_axis',(0.,-0.13147778146049,0.991319117631768));
#1995=DIRECTION('center_axis',(0.,0.999879786123581,-0.0155052668942604));
#1996=DIRECTION('ref_axis',(0.,0.0155052668942604,0.999879786123581));
#1997=DIRECTION('center_axis',(1.22464679914735E-15,1.,0.));
#1998=DIRECTION('ref_axis',(0.,0.,1.));
#2566=CARTESIAN_POINT('',(0.,0.,0.));
#2567=CARTESIAN_POINT('Ctrl Pts',(56.6181736442213,-16.9999774720125,50.2376372405532));
#2568=CARTESIAN_POINT('Ctrl Pts',(56.6181736442213,-17.5445585268313,50.1654099348961));
#2569=CARTESIAN_POINT('Ctrl Pts',(56.6181736442213,-18.5450363459383,49.9971956031968));
#2570=CARTESIAN_POINT('Ctrl Pts',(56.6181736442213,-19.7685844487136,49.493904422604));
#2571=CARTESIAN_POINT('Ctrl Pts',(56.6181736442213,-20.6981100416586,48.489204295438));
#2572=CARTESIAN_POINT('Ctrl Pts',(56.6181736442214,-21.5561871796402,46.50222984823));
#2573=CARTESIAN_POINT('Ctrl Pts',(56.6181736442213,-21.8921327321723,43.9745858341972));
#2574=CARTESIAN_POINT('Ctrl Pts',(56.6181736442213,-21.8405547289732,41.973830798324));
#2575=CARTESIAN_POINT('Ctrl Pts',(56.6181736442213,-21.7909247107181,41.2895085231153));
#2576=CARTESIAN_POINT('Ctrl Pts',(56.618157657027,-16.9607330396014,49.9417411912163));
#2577=CARTESIAN_POINT('Ctrl Pts',(56.618157657027,-17.4971627471983,49.8705949915618));
#2578=CARTESIAN_POINT('Ctrl Pts',(56.6181576570271,-18.4805860762608,49.7024575220591));
#2579=CARTESIAN_POINT('Ctrl Pts',(56.6181576570271,-19.5946720652724,49.2381096635961));
#2580=CARTESIAN_POINT('Ctrl Pts',(56.6181576570271,-20.4358764482362,48.3351593148684));
#2581=CARTESIAN_POINT('Ctrl Pts',(56.6181576570271,-21.2635356262042,46.4375753069283));
#2582=CARTESIAN_POINT('Ctrl Pts',(56.618157657027,-21.5933664996061,43.9574760043368));
#2583=CARTESIAN_POINT('Ctrl Pts',(56.618157657027,-21.5421903626094,41.9863338279172));
#2584=CARTESIAN_POINT('Ctrl Pts',(56.618157657027,-21.4932194344719,41.3110994004402));
#2585=CARTESIAN_POINT('Ctrl Pts',(56.905319880527,-16.8821224243696,49.3490311160804));
#2586=CARTESIAN_POINT('Ctrl Pts',(56.905319880527,-17.402249022489,49.2800471834769));
#2587=CARTESIAN_POINT('Ctrl Pts',(56.9053198805271,-18.351402212785,49.1122156518553));
#2588=CARTESIAN_POINT('Ctrl Pts',(56.9053198805271,-19.2464726950456,48.7258501952951));
#2589=CARTESIAN_POINT('Ctrl Pts',(56.905319880527,-19.9109000058981,48.0265380482217));
#2590=CARTESIAN_POINT('Ctrl Pts',(56.9053198805271,-20.6776200693149,46.3078832788634));
#2591=CARTESIAN_POINT('Ctrl Pts',(56.905319880527,-20.995035487576,43.9231272443799));
#2592=CARTESIAN_POINT('Ctrl Pts',(56.905319880527,-20.9445380069861,42.0114064070899));
#2593=CARTESIAN_POINT('Ctrl Pts',(56.905319880527,-20.896885292642,41.3543481377929));
#2594=CARTESIAN_POINT('Ctrl Pts',(57.8731003937659,-16.8534555622595,49.1328880679052));
#2595=CARTESIAN_POINT('Ctrl Pts',(57.8731003937659,-17.3675474908954,49.0647045082001));
#2596=CARTESIAN_POINT('Ctrl Pts',(57.873100393766,-18.3045926185379,48.8964381348405));
#2597=CARTESIAN_POINT('Ctrl Pts',(57.873100393766,-19.1189021385899,48.5386005456125));
#2598=CARTESIAN_POINT('Ctrl Pts',(57.873100393766,-19.7183632902904,47.914185411008));
#2599=CARTESIAN_POINT('Ctrl Pts',(57.873100393766,-20.4628924782868,46.2612442706814));
#2600=CARTESIAN_POINT('Ctrl Pts',(57.8731003937659,-20.7763812483859,43.9108746314944));
#2601=CARTESIAN_POINT('Ctrl Pts',(57.8731003937659,-20.7265854309009,42.0204498982018));
#2602=CARTESIAN_POINT('Ctrl Pts',(57.8731003937659,-20.6794206593362,41.370119615811));
#2603=CARTESIAN_POINT('Ctrl Pts',(58.6517637674637,-16.9346108560101,49.7447845670574));
#2604=CARTESIAN_POINT('Ctrl Pts',(58.6517637674637,-17.4656187961995,49.6743574516389));
#2605=CARTESIAN_POINT('Ctrl Pts',(58.6517637674638,-18.4376727944556,49.5062955564888));
#2606=CARTESIAN_POINT('Ctrl Pts',(58.6517637674638,-19.478937649954,49.0678654289268));
#2607=CARTESIAN_POINT('Ctrl Pts',(58.6517637674637,-20.2613753689088,48.2326141213349));
#2608=CARTESIAN_POINT('Ctrl Pts',(58.6517637674638,-21.0687860903838,46.3945101552329));
#2609=CARTESIAN_POINT('Ctrl Pts',(58.6517637674637,-21.3945200169302,43.9460750151473));
#2610=CARTESIAN_POINT('Ctrl Pts',(58.6517637674637,-21.3435910811886,41.9946606461063));
#2611=CARTESIAN_POINT('Ctrl Pts',(58.6517637674637,-21.2950585386603,41.3254708877245));
#2612=CARTESIAN_POINT('Ctrl Pts',(58.6489192212011,-17.0652276031362,50.7296116387549));
#2613=CARTESIAN_POINT('Ctrl Pts',(58.6489192212011,-17.6233774657808,50.6555847140666));
#2614=CARTESIAN_POINT('Ctrl Pts',(58.6489192212011,-18.6521419321212,50.4873396881221));
#2615=CARTESIAN_POINT('Ctrl Pts',(58.6489192212011,-20.0578469197985,49.9192830095945));
#2616=CARTESIAN_POINT('Ctrl Pts',(58.6489192212011,-21.1343096540523,48.7452945362702));
#2617=CARTESIAN_POINT('Ctrl Pts',(58.6489192212011,-22.0429558645062,46.6096118224168));
#2618=CARTESIAN_POINT('Ctrl Pts',(58.648919221201,-22.3889612643844,44.002985085501));
#2619=CARTESIAN_POINT('Ctrl Pts',(58.6489192212011,-22.3366343831035,41.9530602347304));
#2620=CARTESIAN_POINT('Ctrl Pts',(58.6489192212011,-22.2859072373551,41.2536102443029));
#2621=CARTESIAN_POINT('Ctrl Pts',(57.8740741606582,-17.146943550959,51.3457353700218));
#2622=CARTESIAN_POINT('Ctrl Pts',(57.8740741606582,-17.7220209683685,51.2694633586541));
#2623=CARTESIAN_POINT('Ctrl Pts',(57.8740741606583,-18.7864945136736,51.1007807270187));
#2624=CARTESIAN_POINT('Ctrl Pts',(57.8740741606583,-20.4196713292811,50.4516808476432));
#2625=CARTESIAN_POINT('Ctrl Pts',(57.8740741606582,-21.6797846595826,49.0661492002334));
#2626=CARTESIAN_POINT('Ctrl Pts',(57.8740741606583,-22.6517841905471,46.7445705314164));
#2627=CARTESIAN_POINT('Ctrl Pts',(57.8740741606582,-23.0108269945255,44.0387505309463));
#2628=CARTESIAN_POINT('Ctrl Pts',(57.8740741606582,-22.9578940458401,41.9269754002992));
#2629=CARTESIAN_POINT('Ctrl Pts',(57.8740741606582,-22.9057981957835,41.2086530644807));
#2630=CARTESIAN_POINT('Ctrl Pts',(56.9054158036926,-17.1175890188362,51.1244074121021));
#2631=CARTESIAN_POINT('Ctrl Pts',(56.9054158036926,-17.6866237002869,51.0489368434824));
#2632=CARTESIAN_POINT('Ctrl Pts',(56.9054158036927,-18.7381038308501,50.8806441386817));
#2633=CARTESIAN_POINT('Ctrl Pts',(56.9054158036927,-20.2899469956927,50.2606187493429));
#2634=CARTESIAN_POINT('Ctrl Pts',(56.9054158036927,-21.4843015664325,48.9508079316389));
#2635=CARTESIAN_POINT('Ctrl Pts',(56.9054158036927,-22.4335293899311,46.6958105266729));
#2636=CARTESIAN_POINT('Ctrl Pts',(56.9054158036926,-22.7876328829734,44.0257862235421));
#2637=CARTESIAN_POINT('Ctrl Pts',(56.9054158036926,-22.7347242051687,41.9363882295308));
#2638=CARTESIAN_POINT('Ctrl Pts',(56.9054158036926,-22.6831169501192,41.2248028738434));
#2639=CARTESIAN_POINT('Ctrl Pts',(56.6181896314156,-17.0392219044236,50.5335332898902));
#2640=CARTESIAN_POINT('Ctrl Pts',(56.6181896314156,-17.5919543064643,50.4602248782303));
#2641=CARTESIAN_POINT('Ctrl Pts',(56.6181896314156,-18.6094866156158,50.2919336843345));
#2642=CARTESIAN_POINT('Ctrl Pts',(56.6181896314156,-19.9424968321547,49.749699181612));
#2643=CARTESIAN_POINT('Ctrl Pts',(56.6181896314156,-20.960343635081,48.6432492760075));
#2644=CARTESIAN_POINT('Ctrl Pts',(56.6181896314156,-21.8488387330763,46.5668843895315));
#2645=CARTESIAN_POINT('Ctrl Pts',(56.6181896314156,-22.1908989647385,43.9916956640576));
#2646=CARTESIAN_POINT('Ctrl Pts',(56.6181896314156,-22.1389190953369,41.9613277687308));
#2647=CARTESIAN_POINT('Ctrl Pts',(56.6181896314156,-22.0886299869643,41.2679176457904));
#2648=CARTESIAN_POINT('Ctrl Pts',(56.6181736442213,-16.9999774720125,50.2376372405532));
#2649=CARTESIAN_POINT('Ctrl Pts',(56.6181736442213,-17.5445585268313,50.1654099348961));
#2650=CARTESIAN_POINT('Ctrl Pts',(56.6181736442213,-18.5450363459383,49.9971956031968));
#2651=CARTESIAN_POINT('Ctrl Pts',(56.6181736442213,-19.7685844487136,49.493904422604));
#2652=CARTESIAN_POINT('Ctrl Pts',(56.6181736442213,-20.6981100416586,48.489204295438));
#2653=CARTESIAN_POINT('Ctrl Pts',(56.6181736442214,-21.5561871796402,46.50222984823));
#2654=CARTESIAN_POINT('Ctrl Pts',(56.6181736442213,-21.8921327321723,43.9745858341972));
#2655=CARTESIAN_POINT('Ctrl Pts',(56.6181736442213,-21.8405547289732,41.973830798324));
#2656=CARTESIAN_POINT('Ctrl Pts',(56.6181736442213,-21.7909247107181,41.2895085231153));
#2657=CARTESIAN_POINT('',(56.6181736442213,-17.1499912781959,50.2172610306738));
#2658=CARTESIAN_POINT('',(57.0353819609965,-17.1500000599476,49.3968517751723));
#2659=CARTESIAN_POINT('Ctrl Pts',(56.6181736442213,-17.1499840472465,50.217262037498));
#2660=CARTESIAN_POINT('Ctrl Pts',(56.618171311048,-17.1500032058279,50.1732731599044));
#2661=CARTESIAN_POINT('Ctrl Pts',(56.6212228953305,-17.1500224012018,50.129369785685));
#2662=CARTESIAN_POINT('Ctrl Pts',(56.6271463571439,-17.1500372451356,50.0858125023058));
#2663=CARTESIAN_POINT('Ctrl Pts',(56.6332115081151,-17.1500524441361,50.0412133290673));
#2664=CARTESIAN_POINT('Ctrl Pts',(56.6422878813441,-17.150062913866,49.9969759001799));
#2665=CARTESIAN_POINT('Ctrl Pts',(56.6542338215383,-17.1500673466086,49.9533857272418));
#2666=CARTESIAN_POINT('Ctrl Pts',(56.6609755223862,-17.1500698482305,49.9287855784817));
#2667=CARTESIAN_POINT('Ctrl Pts',(56.6686320958241,-17.1500705022331,49.9043917713018));
#2668=CARTESIAN_POINT('Ctrl Pts',(56.6771847748605,-17.1500698498811,49.8802584871326));
#2669=CARTESIAN_POINT('Ctrl Pts',(56.6922879026331,-17.1500686978965,49.8376416564502));
#2670=CARTESIAN_POINT('Ctrl Pts',(56.7100899268355,-17.1500625613245,49.7960977151437));
#2671=CARTESIAN_POINT('Ctrl Pts',(56.7304257232293,-17.1500505789465,49.755903064599));
#2672=CARTESIAN_POINT('Ctrl Pts',(56.7505173013739,-17.1500387404682,49.7161911228205));
#2673=CARTESIAN_POINT('Ctrl Pts',(56.7730827717305,-17.1500210684331,49.6777952356117));
#2674=CARTESIAN_POINT('Ctrl Pts',(56.7980079196547,-17.1500018092014,49.6410021939523));
#2675=CARTESIAN_POINT('Ctrl Pts',(56.8213558952837,-17.1499837686235,49.6065372815436));
#2676=CARTESIAN_POINT('Ctrl Pts',(56.8467750941849,-17.1499642905174,49.5734782555144));
#2677=CARTESIAN_POINT('Ctrl Pts',(56.8742014205842,-17.1499524705361,49.5420892426593));
#2678=CARTESIAN_POINT('Ctrl Pts',(56.9034936336824,-17.1499398464098,49.5085647508953));
#2679=CARTESIAN_POINT('Ctrl Pts',(56.934889227382,-17.1499343605014,49.47715818171));
#2680=CARTESIAN_POINT('Ctrl Pts',(56.9682642728882,-17.1499494612514,49.448150109619));
#2681=CARTESIAN_POINT('Ctrl Pts',(56.9769834915822,-17.149953406317,49.4405717611669));
#2682=CARTESIAN_POINT('Ctrl Pts',(56.9858380206297,-17.1499587848582,49.4331572880387));
#2683=CARTESIAN_POINT('Ctrl Pts',(56.9948260768585,-17.1499659012595,49.425912102012));
#2684=CARTESIAN_POINT('Ctrl Pts',(57.0078460491693,-17.1499762099788,49.4154168270545));
#2685=CARTESIAN_POINT('Ctrl Pts',(57.0211461904777,-17.1499901607879,49.4052767435268));
#2686=CARTESIAN_POINT('Ctrl Pts',(57.0347099858223,-17.1500065726219,49.3954939610427));
#2687=CARTESIAN_POINT('',(56.6189035487885,-17.,50.237807097577));
#2688=CARTESIAN_POINT('Ctrl Pts',(57.03538814639,-17.1499999999997,49.3968642735726));
#2689=CARTESIAN_POINT('Ctrl Pts',(56.9904204252509,-17.1349950871205,49.4317323019518));
#2690=CARTESIAN_POINT('Ctrl Pts',(56.9448496571703,-17.1213415050968,49.4725236057591));
#2691=CARTESIAN_POINT('Ctrl Pts',(56.8147498453777,-17.0836252031835,49.6135720251987));
#2692=CARTESIAN_POINT('Ctrl Pts',(56.7451823103795,-17.0646703473624,49.7221064004491));
#2693=CARTESIAN_POINT('Ctrl Pts',(56.6485334490992,-17.0307910857937,49.9593883702037));
#2694=CARTESIAN_POINT('Ctrl Pts',(56.6221206393291,-17.0163863096898,50.0856669992656));
#2695=CARTESIAN_POINT('Ctrl Pts',(56.6189955671074,-17.0017177174059,50.2217783826396));
#2696=CARTESIAN_POINT('Ctrl Pts',(56.6189035487885,-17.0008574567801,50.2297924478132));
#2697=CARTESIAN_POINT('Ctrl Pts',(56.6189035487885,-17.,50.237807097577));
#2698=CARTESIAN_POINT('',(58.6189035487885,-17.,50.237807097577));
#2699=CARTESIAN_POINT('Origin',(57.6189035487885,-17.,50.237807097577));
#2700=CARTESIAN_POINT('Origin',(57.6189035487885,-17.,50.237807097577));
#2701=CARTESIAN_POINT('',(56.6466073920881,-17.1499031620603,50.4512837654741));
#2702=CARTESIAN_POINT('Ctrl Pts',(56.6181736442213,-16.9999774720125,50.2376372405533));
#2703=CARTESIAN_POINT('Ctrl Pts',(56.6181740497314,-17.004940043061,50.2446163905992));
#2704=CARTESIAN_POINT('Ctrl Pts',(56.6182668383978,-17.0098929123044,50.2516016942287));
#2705=CARTESIAN_POINT('Ctrl Pts',(56.6184515899688,-17.0148373029502,50.2585915972787));
#2706=CARTESIAN_POINT('Ctrl Pts',(56.6195366065838,-17.0438749234153,50.2996421870056));
#2707=CARTESIAN_POINT('Ctrl Pts',(56.6237844714869,-17.0725006077051,50.3406683752586));
#2708=CARTESIAN_POINT('Ctrl Pts',(56.6310549101252,-17.1009322593977,50.3813635864379));
#2709=CARTESIAN_POINT('Ctrl Pts',(56.6352421205432,-17.1173066920959,50.4048008810347));
#2710=CARTESIAN_POINT('Ctrl Pts',(56.6404328338326,-17.133616698542,50.4281281830798));
#2711=CARTESIAN_POINT('Ctrl Pts',(56.6466073920881,-17.1499031620603,50.4512837654741));
#2712=CARTESIAN_POINT('Ctrl Pts',(56.6466073920881,-17.1499031620601,50.4512837654741));
#2713=CARTESIAN_POINT('Ctrl Pts',(56.6362214282127,-17.1499120260523,50.4085673066142));
#2714=CARTESIAN_POINT('Ctrl Pts',(56.628577159635,-17.1499259151824,50.3652197513392));
#2715=CARTESIAN_POINT('Ctrl Pts',(56.6238417275253,-17.1499421537733,50.3214930341557));
#2716=CARTESIAN_POINT('Ctrl Pts',(56.6219795567511,-17.1499485394692,50.3042978526174));
#2717=CARTESIAN_POINT('Ctrl Pts',(56.62056775721,-17.1499553023441,50.2870439950997));
#2718=CARTESIAN_POINT('Ctrl Pts',(56.6196187380674,-17.1499623634815,50.2697468149321));
#2719=CARTESIAN_POINT('Ctrl Pts',(56.618658721881,-17.1499695064421,50.2522491985049));
#2720=CARTESIAN_POINT('Ctrl Pts',(56.6181745717269,-17.1499766632751,50.2347488876625));
#2721=CARTESIAN_POINT('Ctrl Pts',(56.6181736442213,-17.1499840472466,50.2172620374986));
#2722=CARTESIAN_POINT('',(56.6189035487885,-21.7910956063159,41.2894961290256));
#2723=CARTESIAN_POINT('Ctrl Pts',(56.6181736442213,-17.1499912781959,50.2172610306739));
#2724=CARTESIAN_POINT('Ctrl Pts',(56.6181736442213,-17.6367273439312,50.1494886908499));
#2725=CARTESIAN_POINT('Ctrl Pts',(56.6181736442213,-18.5827705834998,49.981674097399));
#2726=CARTESIAN_POINT('Ctrl Pts',(56.6181736442213,-19.7685844487136,49.493904422604));
#2727=CARTESIAN_POINT('Ctrl Pts',(56.6181736442213,-20.6981100416586,48.489204295438));
#2728=CARTESIAN_POINT('Ctrl Pts',(56.6181736442214,-21.5561871796402,46.50222984823));
#2729=CARTESIAN_POINT('Ctrl Pts',(56.6181736442213,-21.8921327321723,43.9745858341972));
#2730=CARTESIAN_POINT('Ctrl Pts',(56.6181736442213,-21.8405547289732,41.973830798324));
#2731=CARTESIAN_POINT('Ctrl Pts',(56.6181736442213,-21.7909247107181,41.2895085231153));
#2732=CARTESIAN_POINT('Origin',(57.6189035487885,-21.7910956063159,41.2894961290256));
#2733=CARTESIAN_POINT('Ctrl Pts',(58.6167627387145,-17.1602658348517,50.2165486526461));
#2734=CARTESIAN_POINT('Ctrl Pts',(58.643008473399,-16.178033900518,50.3468677070468));
#2735=CARTESIAN_POINT('Ctrl Pts',(58.2035873080419,-14.2013435692345,50.6075058158481));
#2736=CARTESIAN_POINT('Ctrl Pts',(56.2225937043736,-11.897451182557,50.9984629790502));
#2737=CARTESIAN_POINT('Ctrl Pts',(53.3892837467024,-10.8009462068176,51.3894201422522));
#2738=CARTESIAN_POINT('Ctrl Pts',(50.3736273245558,-11.1706588511001,51.7803773054543));
#2739=CARTESIAN_POINT('Ctrl Pts',(47.8891338131767,-12.9193891815025,52.1713344686563));
#2740=CARTESIAN_POINT('Ctrl Pts',(46.523451423545,-15.6333553665913,52.5622916318584));
#2741=CARTESIAN_POINT('Ctrl Pts',(46.599664491672,-18.6706201350726,52.9532487950604));
#2742=CARTESIAN_POINT('Ctrl Pts',(48.0997310899548,-21.3126898076219,53.3442059582625));
#2743=CARTESIAN_POINT('Ctrl Pts',(50.66881515933,-22.9345914086011,53.7351631214646));
#2744=CARTESIAN_POINT('Ctrl Pts',(53.6991939529023,-23.1526568531196,54.1261202846665));
#2745=CARTESIAN_POINT('Ctrl Pts',(56.47402923455,-21.9153050002011,54.5170774478686));
#2746=CARTESIAN_POINT('Ctrl Pts',(58.3369298825998,-19.5152317078047,54.9080346110706));
#2747=CARTESIAN_POINT('Ctrl Pts',(58.8472248890723,-16.5201776181574,55.2989917742727));
#2748=CARTESIAN_POINT('Ctrl Pts',(57.8842032458303,-13.6386259892673,55.6899489374747));
#2749=CARTESIAN_POINT('Ctrl Pts',(55.6756688973336,-11.5522113011612,56.0809061006768));
#2750=CARTESIAN_POINT('Ctrl Pts',(52.7440531658162,-10.7544773055472,56.4718632638789));
#2751=CARTESIAN_POINT('Ctrl Pts',(49.7828331520566,-11.4341289248563,56.8628204270809));
#2752=CARTESIAN_POINT('Ctrl Pts',(47.4924888644779,-13.430393772254,57.253777590283));
#2753=CARTESIAN_POINT('Ctrl Pts',(46.4148038926073,-16.271053097522,57.644734753485));
#2754=CARTESIAN_POINT('Ctrl Pts',(46.8047058599946,-19.2841456537754,58.035691916687));
#2755=CARTESIAN_POINT('Ctrl Pts',(48.5699630065106,-21.7569209176924,58.4266490798891));
#2756=CARTESIAN_POINT('Ctrl Pts',(51.293001714916,-23.1044410439156,58.8176062430911));
#2757=CARTESIAN_POINT('Ctrl Pts',(54.3296840336396,-23.0079485903805,59.2085634062931));
#2758=CARTESIAN_POINT('Ctrl Pts',(56.9616792526266,-21.4902689583137,59.5995205694953));
#2759=CARTESIAN_POINT('Ctrl Pts',(58.5663858627843,-18.9104110177176,59.9904777326972));
#2760=CARTESIAN_POINT('Ctrl Pts',(58.7642086619611,-15.8786431442651,60.3814348958993));
#2761=CARTESIAN_POINT('Ctrl Pts',(57.5083524385236,-13.112133530256,60.7723920591013));
#2762=CARTESIAN_POINT('Ctrl Pts',(55.095891432692,-11.2653032203185,61.1633492223034));
#2763=CARTESIAN_POINT('Ctrl Pts',(52.0974960818944,-10.77502205744,61.5543063855054));
#2764=CARTESIAN_POINT('Ctrl Pts',(49.2224402696388,-11.7572666169945,61.9452635487075));
#2765=CARTESIAN_POINT('Ctrl Pts',(47.1508217691292,-13.9796858138845,62.3362207119095));
#2766=CARTESIAN_POINT('Ctrl Pts',(46.3726843294707,-16.9165638200946,62.7271778751116));
#2767=CARTESIAN_POINT('Ctrl Pts',(47.0720972607971,-19.8731787510337,63.1181350383136));
#2768=CARTESIAN_POINT('Ctrl Pts',(49.0836136263508,-22.1501399297692,63.5090922015157));
#2769=CARTESIAN_POINT('Ctrl Pts',(51.9314069064712,-23.2088295594817,63.9000493647177));
#2770=CARTESIAN_POINT('Ctrl Pts',(54.9418283114199,-22.7988133854305,64.2910065279198));
#2771=CARTESIAN_POINT('Ctrl Pts',(57.4027591806895,-21.0170812071728,64.6819636911218));
#2772=CARTESIAN_POINT('Ctrl Pts',(58.7320634746702,-18.2851038294562,65.0729208543239));
#2773=CARTESIAN_POINT('Ctrl Pts',(58.6152927272196,-15.2491336565274,65.4638780175259));
#2774=CARTESIAN_POINT('Ctrl Pts',(57.080069193516,-12.6273329394813,65.854835180728));
#2775=CARTESIAN_POINT('Ctrl Pts',(54.4895517737208,-11.039891666206,66.24579234393));
#2776=CARTESIAN_POINT('Ctrl Pts',(51.4565303556175,-10.8623209035087,66.636749507132));
#2777=CARTESIAN_POINT('Ctrl Pts',(48.6984696589939,-12.1366252202991,67.0277066703341));
#2778=CARTESIAN_POINT('Ctrl Pts',(46.8677921271795,-14.5613664587978,67.4186638335361));
#2779=CARTESIAN_POINT('Ctrl Pts',(46.3975466451333,-17.5629692778492,67.8096209967382));
#2780=CARTESIAN_POINT('Ctrl Pts',(47.3989703241477,-20.431401064721,68.2005781599402));
#2781=CARTESIAN_POINT('Ctrl Pts',(49.6351752376468,-22.4881309646939,68.5915353231423));
#2782=CARTESIAN_POINT('Ctrl Pts',(52.5771845274374,-23.2466371494448,68.9824924863443));
#2783=CARTESIAN_POINT('Ctrl Pts',(55.529062504339,-22.5274940937726,69.3734496495464));
#2784=CARTESIAN_POINT('Ctrl Pts',(57.7925390093781,-20.5008159421237,69.7644068127484));
#2785=CARTESIAN_POINT('Ctrl Pts',(58.8321860911263,-17.6460157002987,70.1553639759505));
#2786=CARTESIAN_POINT('Ctrl Pts',(58.4020739661194,-14.6383997751071,70.5463211391525));
#2787=CARTESIAN_POINT('Ctrl Pts',(56.6039462958005,-12.189422944957,70.9372783023545));
#2788=CARTESIAN_POINT('Ctrl Pts',(53.8631519513258,-10.8783940324256,71.3282354655566));
#2789=CARTESIAN_POINT('Ctrl Pts',(50.8280296619087,-11.0154373062825,71.7191926287586));
#2790=CARTESIAN_POINT('Ctrl Pts',(48.2165396770217,-12.5681374761835,72.1101497919607));
#2791=CARTESIAN_POINT('Ctrl Pts',(46.6464360547185,-15.1691962162198,72.5011069551627));
#2792=CARTESIAN_POINT('Ctrl Pts',(46.4891218839111,-18.2033415583671,72.8920641183648));
#2793=CARTESIAN_POINT('Ctrl Pts',(47.7818243197045,-20.9528181004838,73.2830212815669));
#2794=CARTESIAN_POINT('Ctrl Pts',(50.2187210719051,-22.7672877187656,73.6739784447688));
#2795=CARTESIAN_POINT('Ctrl Pts',(53.2234261185118,-23.2174195646428,74.0649356079709));
#2796=CARTESIAN_POINT('Ctrl Pts',(56.085013860659,-22.196986288013,74.4558927711729));
#2797=CARTESIAN_POINT('Ctrl Pts',(58.1268398486099,-19.9468301996286,74.846849934375));
#2798=CARTESIAN_POINT('Ctrl Pts',(58.6189035487885,-17.9825825214271,75.1074880431764));
#2799=CARTESIAN_POINT('Ctrl Pts',(58.6189035487885,-17.,75.237807097577));
#2800=CARTESIAN_POINT('Ctrl Pts',(58.6167627387145,-17.1602658348517,49.9173493523042));
#2801=CARTESIAN_POINT('Ctrl Pts',(58.6430203769705,-16.1775884160157,50.0476684067049));
#2802=CARTESIAN_POINT('Ctrl Pts',(58.2038523387604,-14.2013635408179,50.3083065155063));
#2803=CARTESIAN_POINT('Ctrl Pts',(56.2227257314925,-11.8971076065531,50.6992636787083));
#2804=CARTESIAN_POINT('Ctrl Pts',(53.3893294286404,-10.8006864834937,51.0902208419104));
#2805=CARTESIAN_POINT('Ctrl Pts',(50.3735128366562,-11.1703590497448,51.4811780051124));
#2806=CARTESIAN_POINT('Ctrl Pts',(47.8889087174286,-12.9192014916732,51.8721351683145));
#2807=CARTESIAN_POINT('Ctrl Pts',(46.5231569839263,-15.6332855689878,52.2630923315165));
#2808=CARTESIAN_POINT('Ctrl Pts',(46.5993755176917,-18.6707023464517,52.6540494947186));
#2809=CARTESIAN_POINT('Ctrl Pts',(48.0995134617038,-21.3128963800501,53.0450066579206));
#2810=CARTESIAN_POINT('Ctrl Pts',(50.6687214804671,-22.9348772546735,53.4359638211227));
#2811=CARTESIAN_POINT('Ctrl Pts',(53.6992458585534,-23.1529526054874,53.8269209843247));
#2812=CARTESIAN_POINT('Ctrl Pts',(56.4742146877366,-21.9155415067111,54.2178781475268));
#2813=CARTESIAN_POINT('Ctrl Pts',(58.3372049022515,-19.5153526485723,54.6088353107288));
#2814=CARTESIAN_POINT('Ctrl Pts',(58.8475244706438,-16.5201545573878,54.9997924739308));
#2815=CARTESIAN_POINT('Ctrl Pts',(57.8844564990454,-13.6384643020619,55.3907496371328));
#2816=CARTESIAN_POINT('Ctrl Pts',(55.6758159259031,-11.5519492717804,55.7817068003349));
#2817=CARTESIAN_POINT('Ctrl Pts',(52.7440591848512,-10.7541769002508,56.172663963537));
#2818=CARTESIAN_POINT('Ctrl Pts',(49.7826967401103,-11.4338612127674,56.563621126739));
#2819=CARTESIAN_POINT('Ctrl Pts',(47.4922422888612,-13.4302220773222,56.9545782899411));
#2820=CARTESIAN_POINT('Ctrl Pts',(46.4145054815723,-16.2710180360713,57.3455354531431));
#2821=CARTESIAN_POINT('Ctrl Pts',(46.8044262027827,-19.2842555188512,57.7364926163451));
#2822=CARTESIAN_POINT('Ctrl Pts',(48.5697682564663,-21.7571497209455,58.1274497795472));
#2823=CARTESIAN_POINT('Ctrl Pts',(51.2929379403373,-23.1047346615051,58.5184069427492));
#2824=CARTESIAN_POINT('Ctrl Pts',(54.3297663204998,-23.0082375668037,58.9093641059513));
#2825=CARTESIAN_POINT('Ctrl Pts',(56.9618881358633,-21.4904849358282,59.3003212691533));
#2826=CARTESIAN_POINT('Ctrl Pts',(58.5666719308314,-18.9105029066094,59.6912784323554));
#2827=CARTESIAN_POINT('Ctrl Pts',(58.7645042450895,-15.878589208103,60.0822355955574));
#2828=CARTESIAN_POINT('Ctrl Pts',(57.5085876162038,-13.1119465277051,60.4731927587594));
#2829=CARTESIAN_POINT('Ctrl Pts',(55.0960105733717,-11.2650273870465,60.8641499219615));
#2830=CARTESIAN_POINT('Ctrl Pts',(52.0974710027084,-10.7747226421268,61.2551070851635));
#2831=CARTESIAN_POINT('Ctrl Pts',(49.2222769030974,-11.7570144466779,61.6460642483656));
#2832=CARTESIAN_POINT('Ctrl Pts',(47.1505587597765,-13.9795405397443,62.0370214115676));
#2833=CARTESIAN_POINT('Ctrl Pts',(46.3723838924729,-16.9165598068964,62.4279785747697));
#2834=CARTESIAN_POINT('Ctrl Pts',(47.0718304648731,-19.8733169481042,62.8189357379717));
#2835=CARTESIAN_POINT('Ctrl Pts',(49.0834435823845,-22.1503876464318,63.2098929011738));
#2836=CARTESIAN_POINT('Ctrl Pts',(51.9313738385592,-23.2091281980736,63.6008500643758));
#2837=CARTESIAN_POINT('Ctrl Pts',(54.9419400418151,-22.7990923026481,63.9918072275779));
#2838=CARTESIAN_POINT('Ctrl Pts',(57.4029892794379,-21.0172744248255,64.3827643907799));
#2839=CARTESIAN_POINT('Ctrl Pts',(58.7323575116467,-18.2851656416866,64.773721553982));
#2840=CARTESIAN_POINT('Ctrl Pts',(58.6155811476388,-15.2490494415775,65.164678717184));
#2841=CARTESIAN_POINT('Ctrl Pts',(57.0802837711922,-12.6271226185024,65.5556358803861));
#2842=CARTESIAN_POINT('Ctrl Pts',(54.4896417500622,-11.0396049908522,65.9465930435881));
#2843=CARTESIAN_POINT('Ctrl Pts',(51.4564744466051,-10.8620256872015,66.3375502067901));
#2844=CARTESIAN_POINT('Ctrl Pts',(48.6982810899941,-12.1363912967204,66.7285073699922));
#2845=CARTESIAN_POINT('Ctrl Pts',(46.8675155043528,-14.5612491630059,67.1194645331942));
#2846=CARTESIAN_POINT('Ctrl Pts',(46.3972474040464,-17.5629963559409,67.5104216963963));
#2847=CARTESIAN_POINT('Ctrl Pts',(47.3987192503709,-20.4315661121173,67.9013788595984));
#2848=CARTESIAN_POINT('Ctrl Pts',(49.6350317235223,-22.4883949375669,68.2923360228004));
#2849=CARTESIAN_POINT('Ctrl Pts',(52.5771825202072,-23.2469376083305,68.6832931860024));
#2850=CARTESIAN_POINT('Ctrl Pts',(55.5292024813889,-22.527759956937,69.0742503492045));
#2851=CARTESIAN_POINT('Ctrl Pts',(57.7927878534096,-20.5009843362785,69.4652075124065));
#2852=CARTESIAN_POINT('Ctrl Pts',(58.832484949831,-17.6460467549552,69.8561646756086));
#2853=CARTESIAN_POINT('Ctrl Pts',(58.4023521180891,-14.6382862235337,70.2471218388106));
#2854=CARTESIAN_POINT('Ctrl Pts',(56.604138000136,-12.1891914764678,70.6380790020127));
#2855=CARTESIAN_POINT('Ctrl Pts',(53.8632117382902,-10.8780997720332,71.0290361652147));
#2856=CARTESIAN_POINT('Ctrl Pts',(50.8279436516972,-11.015149059947,71.4199933284168));
#2857=CARTESIAN_POINT('Ctrl Pts',(48.2163276441712,-12.5679251643986,71.8109504916188));
#2858=CARTESIAN_POINT('Ctrl Pts',(46.6461493797905,-15.1691063153978,72.2019076548208));
#2859=CARTESIAN_POINT('Ctrl Pts',(46.4888256849871,-18.2034034662982,72.5928648180229));
#2860=CARTESIAN_POINT('Ctrl Pts',(47.781594290893,-20.9529997108187,72.983821981225));
#2861=CARTESIAN_POINT('Ctrl Pts',(50.2185986168693,-22.7675843550681,73.3747791444269));
#2862=CARTESIAN_POINT('Ctrl Pts',(53.2234648466879,-23.2176804155059,73.765736307629));
#2863=CARTESIAN_POINT('Ctrl Pts',(56.0851366634212,-22.1973332680011,74.1566934708311));
#2864=CARTESIAN_POINT('Ctrl Pts',(58.1271053182254,-19.9468173143993,74.5476506340331));
#2865=CARTESIAN_POINT('Ctrl Pts',(58.6189035487885,-17.9830281649358,74.8082887428345));
#2866=CARTESIAN_POINT('Ctrl Pts',(58.6189035487885,-17.,74.9386077972352));
#2867=CARTESIAN_POINT('Ctrl Pts',(58.330235267061,-17.1526096757125,49.3207360155538));
#2868=CARTESIAN_POINT('Ctrl Pts',(58.3552250931434,-16.2173794180463,49.4510550699545));
#2869=CARTESIAN_POINT('Ctrl Pts',(57.9367509801763,-14.3350363953506,49.7116931787559));
#2870=CARTESIAN_POINT('Ctrl Pts',(56.0504162024209,-12.1412690460258,50.1026503419579));
#2871=CARTESIAN_POINT('Ctrl Pts',(53.3524733469576,-11.0971310491503,50.49360750516));
#2872=CARTESIAN_POINT('Ctrl Pts',(50.4809080825804,-11.4491890150081,50.884564668362));
#2873=CARTESIAN_POINT('Ctrl Pts',(48.1151224405566,-13.1143598116086,51.2755218315641));
#2874=CARTESIAN_POINT('Ctrl Pts',(46.8146931916843,-15.6986545556209,51.6664789947661));
#2875=CARTESIAN_POINT('Ctrl Pts',(46.8872644702461,-18.5907973452297,52.0574361579682));
#2876=CARTESIAN_POINT('Ctrl Pts',(48.3156578215541,-21.106629044687,52.4483933211702));
#2877=CARTESIAN_POINT('Ctrl Pts',(50.7619906314754,-22.6510357393524,52.8393504843722));
#2878=CARTESIAN_POINT('Ctrl Pts',(53.6475775376757,-22.8586820898609,53.2303076475743));
#2879=CARTESIAN_POINT('Ctrl Pts',(56.2898307912776,-21.6804510319926,53.6212648107763));
#2880=CARTESIAN_POINT('Ctrl Pts',(58.0637217951495,-19.3950535957025,54.0122219739784));
#2881=CARTESIAN_POINT('Ctrl Pts',(58.5496348325434,-16.5431035947391,54.4031791371804));
#2882=CARTESIAN_POINT('Ctrl Pts',(57.6326264980959,-13.7992329061659,54.7941363003825));
#2883=CARTESIAN_POINT('Ctrl Pts',(55.5296162257536,-11.8125073984122,55.1850934635845));
#2884=CARTESIAN_POINT('Ctrl Pts',(52.7380734998907,-11.0528892445139,55.5760506267866));
#2885=CARTESIAN_POINT('Ctrl Pts',(49.9183409880472,-11.7000670149304,55.9670077899886));
#2886=CARTESIAN_POINT('Ctrl Pts',(47.7374296675502,-13.6009500518754,56.3579649531906));
#2887=CARTESIAN_POINT('Ctrl Pts',(46.7112366327447,-16.3058822813685,56.7489221163927));
#2888=CARTESIAN_POINT('Ctrl Pts',(47.0825090301861,-19.1750088583536,57.1398792795947));
#2889=CARTESIAN_POINT('Ctrl Pts',(48.7634219459444,-21.5296345779364,57.5308364427968));
#2890=CARTESIAN_POINT('Ctrl Pts',(51.3563534880287,-22.8127700060576,57.9217936059988));
#2891=CARTESIAN_POINT('Ctrl Pts',(54.247942705321,-22.7208879753013,58.3127507692009));
#2892=CARTESIAN_POINT('Ctrl Pts',(56.7541808285083,-21.2757232860857,58.7037079324029));
#2893=CARTESIAN_POINT('Ctrl Pts',(58.2822143347599,-18.8191313149124,59.094665095605));
#2894=CARTESIAN_POINT('Ctrl Pts',(58.4705851332158,-15.9322217300148,59.4856222588071));
#2895=CARTESIAN_POINT('Ctrl Pts',(57.2747338939298,-13.2978963282153,59.876579422009));
#2896=CARTESIAN_POINT('Ctrl Pts',(54.9775406088131,-11.5393078260663,60.2675365852111));
#2897=CARTESIAN_POINT('Ctrl Pts',(52.1224090028193,-11.0724523649993,60.6584937484131));
#2898=CARTESIAN_POINT('Ctrl Pts',(49.3847237551472,-12.0077651435671,61.0494509116152));
#2899=CARTESIAN_POINT('Ctrl Pts',(47.4120874732796,-14.1239968436731,61.4404080748173));
#2900=CARTESIAN_POINT('Ctrl Pts',(46.671129548173,-16.920550412317,61.8313652380193));
#2901=CARTESIAN_POINT('Ctrl Pts',(47.3371244328501,-19.7358978726952,62.2223224012214));
#2902=CARTESIAN_POINT('Ctrl Pts',(49.2525302680875,-21.904065531206,62.6132795644234));
#2903=CARTESIAN_POINT('Ctrl Pts',(51.9642555911825,-22.9121708239007,63.0042367276254));
#2904=CARTESIAN_POINT('Ctrl Pts',(54.830838644796,-22.521745279387,63.3951938908275));
#2905=CARTESIAN_POINT('Ctrl Pts',(57.1741858965679,-20.8251445111774,63.7861510540295));
#2906=CARTESIAN_POINT('Ctrl Pts',(58.4399758474222,-18.2237013906414,64.1771082172316));
#2907=CARTESIAN_POINT('Ctrl Pts',(58.3287844224443,-15.3327902927182,64.5680653804336));
#2908=CARTESIAN_POINT('Ctrl Pts',(56.8669140816383,-12.836259576758,64.9590225436357));
#2909=CARTESIAN_POINT('Ctrl Pts',(54.4001719426573,-11.3246664672051,65.3499797068377));
#2910=CARTESIAN_POINT('Ctrl Pts',(51.5120687076471,-11.1555800601186,65.7409368700398));
#2911=CARTESIAN_POINT('Ctrl Pts',(48.8857885327881,-12.3689979403138,66.1318940332418));
#2912=CARTESIAN_POINT('Ctrl Pts',(47.142581026795,-14.6778847068602,66.5228511964439));
#2913=CARTESIAN_POINT('Ctrl Pts',(46.6948039389424,-17.5360705278765,66.9138083596459));
#2914=CARTESIAN_POINT('Ctrl Pts',(47.6483794560206,-20.2674482469155,67.304765522848));
#2915=CARTESIAN_POINT('Ctrl Pts',(49.7777381892181,-22.2259073078542,67.69572268605));
#2916=CARTESIAN_POINT('Ctrl Pts',(52.5791778681548,-22.9481719616671,68.086679849252));
#2917=CARTESIAN_POINT('Ctrl Pts',(55.3900147064866,-22.2633896617156,68.4776370124541));
#2918=CARTESIAN_POINT('Ctrl Pts',(57.5453419915864,-20.3335464704585,68.8685941756561));
#2919=CARTESIAN_POINT('Ctrl Pts',(58.5353145903586,-17.6151489839351,69.2595513388582));
#2920=CARTESIAN_POINT('Ctrl Pts',(58.125753285529,-14.7512373537532,69.6505085020602));
#2921=CARTESIAN_POINT('Ctrl Pts',(56.4135403969614,-12.419272997327,70.0414656652623));
#2922=CARTESIAN_POINT('Ctrl Pts',(53.8037016011131,-11.1708851803488,70.4324228284643));
#2923=CARTESIAN_POINT('Ctrl Pts',(50.9135978412127,-11.3013806098642,70.8233799916664));
#2924=CARTESIAN_POINT('Ctrl Pts',(48.4268852822336,-12.7798923292767,71.2143371548684));
#2925=CARTESIAN_POINT('Ctrl Pts',(46.931801272795,-15.2566726002688,71.6052943180705));
#2926=CARTESIAN_POINT('Ctrl Pts',(46.7820039413394,-18.1458450190503,71.9962514812725));
#2927=CARTESIAN_POINT('Ctrl Pts',(48.012940169097,-20.7639534122315,72.3872086444746));
#2928=CARTESIAN_POINT('Ctrl Pts',(50.3334033635168,-22.4917225082625,72.7781658076765));
#2929=CARTESIAN_POINT('Ctrl Pts',(53.1945402379506,-22.9203571599847,73.1691229708786));
#2930=CARTESIAN_POINT('Ctrl Pts',(55.9194104041682,-21.9486563906518,73.5600801340807));
#2931=CARTESIAN_POINT('Ctrl Pts',(57.8636697937926,-19.8060576175284,73.9510372972827));
#2932=CARTESIAN_POINT('Ctrl Pts',(58.3322738071619,-17.9355640684967,74.2116754060841));
#2933=CARTESIAN_POINT('Ctrl Pts',(58.3322738071619,-17.,74.3419944604848));
#2934=CARTESIAN_POINT('Ctrl Pts',(57.3629302665031,-17.1267627962574,49.1017733081928));
#2935=CARTESIAN_POINT('Ctrl Pts',(57.3836892708566,-16.3498686743689,49.2320923625935));
#2936=CARTESIAN_POINT('Ctrl Pts',(57.0361245100955,-14.7863931213031,49.4927304713948));
#2937=CARTESIAN_POINT('Ctrl Pts',(55.4692526586416,-12.9641262477274,49.8836876345969));
#2938=CARTESIAN_POINT('Ctrl Pts',(53.22823777004,-12.0968409470713,50.2746447977989));
#2939=CARTESIAN_POINT('Ctrl Pts',(50.8429962491044,-12.3892668902023,50.665601961001));
#2940=CARTESIAN_POINT('Ctrl Pts',(48.8778791909101,-13.7724295894674,51.056559124203));
#2941=CARTESIAN_POINT('Ctrl Pts',(47.7976890090763,-15.9190487338459,51.4475162874051));
#2942=CARTESIAN_POINT('Ctrl Pts',(47.8579699218521,-18.3213815491006,51.8384734506071));
#2943=CARTESIAN_POINT('Ctrl Pts',(49.0444517167168,-20.4111338273766,52.2294306138092));
#2944=CARTESIAN_POINT('Ctrl Pts',(51.076475793977,-21.693981325825,52.6203877770112));
#2945=CARTESIAN_POINT('Ctrl Pts',(53.4733622037495,-21.8664607936859,53.0113449402132));
#2946=CARTESIAN_POINT('Ctrl Pts',(55.6681257696359,-20.8877739529222,53.4023021034153));
#2947=CARTESIAN_POINT('Ctrl Pts',(57.1415921405513,-18.9894294095287,53.7932592666173));
#2948=CARTESIAN_POINT('Ctrl Pts',(57.5452113735144,-16.6204831725212,54.1842164298194));
#2949=CARTESIAN_POINT('Ctrl Pts',(56.7835067669695,-14.3413120187973,54.5751735930214));
#2950=CARTESIAN_POINT('Ctrl Pts',(55.0366604743356,-12.6910566059545,54.9661307562235));
#2951=CARTESIAN_POINT('Ctrl Pts',(52.7178909811946,-12.060086717031,55.3570879194255));
#2952=CARTESIAN_POINT('Ctrl Pts',(50.3757058998908,-12.5976590270012,55.7480450826276));
#2953=CARTESIAN_POINT('Ctrl Pts',(48.5641518118953,-14.1766101762591,56.1390022458296));
#2954=CARTESIAN_POINT('Ctrl Pts',(47.711753931384,-16.4234374507423,56.5299594090317));
#2955=CARTESIAN_POINT('Ctrl Pts',(48.0201479605143,-18.8066512616149,56.9209165722337));
#2956=CARTESIAN_POINT('Ctrl Pts',(49.4163829359652,-20.7624996300655,57.3118737354358));
#2957=CARTESIAN_POINT('Ctrl Pts',(51.5701778613603,-21.8283243650465,57.7028308986378));
#2958=CARTESIAN_POINT('Ctrl Pts',(53.9720500594727,-21.7520033946092,58.0937880618398));
#2959=CARTESIAN_POINT('Ctrl Pts',(56.0538338875247,-20.5515905323791,58.4847452250419));
#2960=CARTESIAN_POINT('Ctrl Pts',(57.3230809764613,-18.5110448274855,58.8757023882439));
#2961=CARTESIAN_POINT('Ctrl Pts',(57.4795494613489,-16.1130597233218,59.266659551446));
#2962=CARTESIAN_POINT('Ctrl Pts',(56.486226541364,-13.9248813660636,59.657616714648));
#2963=CARTESIAN_POINT('Ctrl Pts',(54.5780839005581,-12.4641258735578,60.0485738778501));
#2964=CARTESIAN_POINT('Ctrl Pts',(52.2064948846027,-12.0763366447948,60.4395310410521));
#2965=CARTESIAN_POINT('Ctrl Pts',(49.9324616145104,-12.853245669751,60.8304882042542));
#2966=CARTESIAN_POINT('Ctrl Pts',(48.2939092869291,-14.6110742212096,61.2214453674562));
#2967=CARTESIAN_POINT('Ctrl Pts',(47.6784393475473,-16.9340059249544,61.6124025306583));
#2968=CARTESIAN_POINT('Ctrl Pts',(48.2316419214206,-19.2725486033772,62.0033596938603));
#2969=CARTESIAN_POINT('Ctrl Pts',(49.822656300726,-21.0735172847786,62.3943168570624));
#2970=CARTESIAN_POINT('Ctrl Pts',(52.0751261963482,-21.9108907473756,62.7852740202644));
#2971=CARTESIAN_POINT('Ctrl Pts',(54.4562272527764,-21.5865873313883,63.1762311834664));
#2972=CARTESIAN_POINT('Ctrl Pts',(56.4027072648377,-20.1773213844524,63.5671883466685));
#2973=CARTESIAN_POINT('Ctrl Pts',(57.4541241374087,-18.0164563940808,63.9581455098706));
#2974=CARTESIAN_POINT('Ctrl Pts',(57.3617639948527,-15.6151474696354,64.3491026730726));
#2975=CARTESIAN_POINT('Ctrl Pts',(56.1474747355664,-13.5414270108184,64.7400598362746));
#2976=CARTESIAN_POINT('Ctrl Pts',(54.0984978864016,-12.2858359873825,65.1310169994767));
#2977=CARTESIAN_POINT('Ctrl Pts',(51.6995212876628,-12.1453859062227,65.5219741626787));
#2978=CARTESIAN_POINT('Ctrl Pts',(49.5180256247538,-13.1533003961791,65.9129313258808));
#2979=CARTESIAN_POINT('Ctrl Pts',(48.070046216351,-15.0711561206497,66.3038884890828));
#2980=CARTESIAN_POINT('Ctrl Pts',(47.6981042642231,-17.4452820924095,66.6948456522848));
#2981=CARTESIAN_POINT('Ctrl Pts',(48.4901830662541,-19.7140760714731,67.0858028154869));
#2982=CARTESIAN_POINT('Ctrl Pts',(50.2589154680217,-21.3408522196918,67.4767599786889));
#2983=CARTESIAN_POINT('Ctrl Pts',(52.5859057745809,-21.9407947641979,67.867717141891));
#2984=CARTESIAN_POINT('Ctrl Pts',(54.9207017462093,-21.371986594498,68.258674305093));
#2985=CARTESIAN_POINT('Ctrl Pts',(56.7110046880626,-19.7689799587983,68.649631468295));
#2986=CARTESIAN_POINT('Ctrl Pts',(57.5333163950786,-17.5109678879486,69.0405886314972));
#2987=CARTESIAN_POINT('Ctrl Pts',(57.1931180318675,-15.1320858327137,69.4315457946991));
#2988=CARTESIAN_POINT('Ctrl Pts',(55.7708840250745,-13.1950609021638,69.8225029579012));
#2989=CARTESIAN_POINT('Ctrl Pts',(53.6030452317789,-12.15809898931,70.2134601211033));
#2990=CARTESIAN_POINT('Ctrl Pts',(51.2024069407833,-12.2664937492894,70.6044172843053));
#2991=CARTESIAN_POINT('Ctrl Pts',(49.1368417889046,-13.4946061863996,70.9953744475074));
#2992=CARTESIAN_POINT('Ctrl Pts',(47.8949640171512,-15.551920754989,71.3863316107094));
#2993=CARTESIAN_POINT('Ctrl Pts',(47.7705359670016,-17.9517862520598,71.7772887739114));
#2994=CARTESIAN_POINT('Ctrl Pts',(48.7930024502845,-20.1264924093384,72.1682459371135));
#2995=CARTESIAN_POINT('Ctrl Pts',(50.720472730624,-21.5616517814822,72.5592031003155));
#2996=CARTESIAN_POINT('Ctrl Pts',(53.0970522120621,-21.9176855071583,72.9501602635176));
#2997=CARTESIAN_POINT('Ctrl Pts',(55.3604335365829,-21.1105693423597,73.3411174267197));
#2998=CARTESIAN_POINT('Ctrl Pts',(56.975420845832,-19.3308053275606,73.7320745899216));
#2999=CARTESIAN_POINT('Ctrl Pts',(57.3646235473666,-17.7771714179553,73.992712698723));
#3000=CARTESIAN_POINT('Ctrl Pts',(57.3646235473666,-17.,74.1230317531237));
#3001=CARTESIAN_POINT('Ctrl Pts',(56.5845288048375,-17.1059635150217,49.7194456573622));
#3002=CARTESIAN_POINT('Ctrl Pts',(56.6018873807864,-16.4563285234116,49.8497647117628));
#3003=CARTESIAN_POINT('Ctrl Pts',(56.3114727064722,-15.1496120547916,50.1104028205642));
#3004=CARTESIAN_POINT('Ctrl Pts',(55.0016298373768,-13.6261687602616,50.5013599837662));
#3005=CARTESIAN_POINT('Ctrl Pts',(53.1282799464391,-12.9012281808381,50.8923171469683));
#3006=CARTESIAN_POINT('Ctrl Pts',(51.134332727303,-13.145653534561,51.2832743101703));
#3007=CARTESIAN_POINT('Ctrl Pts',(49.491599609735,-14.301920277547,51.6742314733724));
#3008=CARTESIAN_POINT('Ctrl Pts',(48.5886140901663,-16.0963780572031,52.0651886365744));
#3009=CARTESIAN_POINT('Ctrl Pts',(48.6390067154644,-18.1046083068019,52.4561457997765));
#3010=CARTESIAN_POINT('Ctrl Pts',(49.6308444465451,-19.8515330606131,52.8471029629785));
#3011=CARTESIAN_POINT('Ctrl Pts',(51.3295128638488,-20.9239285858085,53.2380601261806));
#3012=CARTESIAN_POINT('Ctrl Pts',(53.3331872710697,-21.0681123227409,53.6290172893826));
#3013=CARTESIAN_POINT('Ctrl Pts',(55.167897437096,-20.2499802915631,54.0199744525847));
#3014=CARTESIAN_POINT('Ctrl Pts',(56.3996399699669,-18.6630612519638,54.4109316157867));
#3015=CARTESIAN_POINT('Ctrl Pts',(56.7370450207677,-16.6827433448981,54.8018887789888));
#3016=CARTESIAN_POINT('Ctrl Pts',(56.1002989102808,-14.7774727769823,55.1928459421908));
#3017=CARTESIAN_POINT('Ctrl Pts',(54.6400247241077,-13.3979436319654,55.5838031053928));
#3018=CARTESIAN_POINT('Ctrl Pts',(52.7016519809952,-12.8704850622985,55.9747602685949));
#3019=CARTESIAN_POINT('Ctrl Pts',(50.7437050045659,-13.3198680297186,56.3657174317969));
#3020=CARTESIAN_POINT('Ctrl Pts',(49.2293384079051,-14.6397904613506,56.756674594999));
#3021=CARTESIAN_POINT('Ctrl Pts',(48.5167773612496,-16.5180231873773,57.147631758201));
#3022=CARTESIAN_POINT('Ctrl Pts',(48.7745790020052,-18.5102680842638,57.5385889214031));
#3023=CARTESIAN_POINT('Ctrl Pts',(49.9417600548431,-20.1452573217946,57.9295460846051));
#3024=CARTESIAN_POINT('Ctrl Pts',(51.7422224933087,-21.0362323067597,58.3205032478071));
#3025=CARTESIAN_POINT('Ctrl Pts',(53.750064848091,-20.9724318776226,58.7114604110092));
#3026=CARTESIAN_POINT('Ctrl Pts',(55.4903296909651,-19.9689480994622,59.1024175742113));
#3027=CARTESIAN_POINT('Ctrl Pts',(56.5513553632931,-18.263156219128,59.4933747374133));
#3028=CARTESIAN_POINT('Ctrl Pts',(56.6821550167432,-16.2585632761502,59.8843319006154));
#3029=CARTESIAN_POINT('Ctrl Pts',(55.8517878422178,-14.4293580465946,60.2752890638173));
#3030=CARTESIAN_POINT('Ctrl Pts',(54.2566781539587,-13.2082411403187,60.6662462270195));
#3031=CARTESIAN_POINT('Ctrl Pts',(52.274150991146,-12.884069171948,61.0572033902214));
#3032=CARTESIAN_POINT('Ctrl Pts',(50.3731754440476,-13.533525395032,61.4481605534236));
#3033=CARTESIAN_POINT('Ctrl Pts',(49.0034294740396,-15.0029801898505,61.8391177166255));
#3034=CARTESIAN_POINT('Ctrl Pts',(48.4889280724435,-16.9448323274048,62.2300748798276));
#3035=CARTESIAN_POINT('Ctrl Pts',(48.9513771400784,-18.8997344416325,62.6210320430297));
#3036=CARTESIAN_POINT('Ctrl Pts',(50.2813838158464,-20.405252179416,63.0119892062317));
#3037=CARTESIAN_POINT('Ctrl Pts',(52.1643334843792,-21.1052535809439,63.4029463694338));
#3038=CARTESIAN_POINT('Ctrl Pts',(54.1548122266959,-20.8341525061532,63.7939035326358));
#3039=CARTESIAN_POINT('Ctrl Pts',(55.7819699972127,-19.6560782274179,64.1848606958379));
#3040=CARTESIAN_POINT('Ctrl Pts',(56.6609007458743,-17.8497055761026,64.5758178590399));
#3041=CARTESIAN_POINT('Ctrl Pts',(56.5836923888842,-15.8423340893094,64.966775022242));
#3042=CARTESIAN_POINT('Ctrl Pts',(55.5686086522617,-14.108809810853,65.357732185444));
#3043=CARTESIAN_POINT('Ctrl Pts',(53.8557687663833,-13.0591999110719,65.748689348646));
#3044=CARTESIAN_POINT('Ctrl Pts',(51.850346984631,-12.9417908241617,66.139646511848));
#3045=CARTESIAN_POINT('Ctrl Pts',(50.0267281458869,-13.7843558051195,66.5306036750501));
#3046=CARTESIAN_POINT('Ctrl Pts',(48.8162913926872,-15.3875851347693,66.9215608382521));
#3047=CARTESIAN_POINT('Ctrl Pts',(48.5053669373851,-17.3722330628012,67.3125180014542));
#3048=CARTESIAN_POINT('Ctrl Pts',(49.1675043184158,-19.2688288307419,67.7034751646563));
#3049=CARTESIAN_POINT('Ctrl Pts',(50.6460741747913,-20.6287305163151,68.0944323278583));
#3050=CARTESIAN_POINT('Ctrl Pts',(52.5913190963785,-21.1302518109333,68.4853894910603));
#3051=CARTESIAN_POINT('Ctrl Pts',(54.5430891561779,-20.6547572603577,68.8763466542624));
#3052=CARTESIAN_POINT('Ctrl Pts',(56.0396908790909,-19.3147256772493,69.2673038174644));
#3053=CARTESIAN_POINT('Ctrl Pts',(56.7271014271941,-17.427143020902,69.6582609806665));
#3054=CARTESIAN_POINT('Ctrl Pts',(56.4427129801899,-15.4385192775656,70.0492181438685));
#3055=CARTESIAN_POINT('Ctrl Pts',(55.25379808591,-13.8192654124519,70.4401753070706));
#3056=CARTESIAN_POINT('Ctrl Pts',(53.4415956497174,-12.9524183994117,70.8311324702726));
#3057=CARTESIAN_POINT('Ctrl Pts',(51.4347848690605,-13.0430305994039,71.2220896334747));
#3058=CARTESIAN_POINT('Ctrl Pts',(49.7080778121442,-14.0696704067362,71.6130467966767));
#3059=CARTESIAN_POINT('Ctrl Pts',(48.6699319114158,-15.7894789045273,72.0040039598788));
#3060=CARTESIAN_POINT('Ctrl Pts',(48.5659154833699,-17.7956465781739,72.3949611230808));
#3061=CARTESIAN_POINT('Ctrl Pts',(49.4206471038287,-19.61358371364,72.7859182862829));
#3062=CARTESIAN_POINT('Ctrl Pts',(51.0319090823161,-20.8133168977984,73.1768754494849));
#3063=CARTESIAN_POINT('Ctrl Pts',(53.0186160188411,-21.1109153094321,73.567832612687));
#3064=CARTESIAN_POINT('Ctrl Pts',(54.9106613632555,-20.436272387398,73.958789775889));
#3065=CARTESIAN_POINT('Ctrl Pts',(56.2607295301239,-18.9483598368167,74.349746939091));
#3066=CARTESIAN_POINT('Ctrl Pts',(56.585944251621,-17.6498668651987,74.6103850478924));
#3067=CARTESIAN_POINT('Ctrl Pts',(56.585944251621,-17.,74.7407041022931));
#3068=CARTESIAN_POINT('Ctrl Pts',(56.5875334327637,-17.1060438002014,50.7124861445407));
#3069=CARTESIAN_POINT('Ctrl Pts',(56.6048933380944,-16.4563590572218,50.8428051989414));
#3070=CARTESIAN_POINT('Ctrl Pts',(56.314007219291,-15.1481902389634,51.1034433077427));
#3071=CARTESIAN_POINT('Ctrl Pts',(55.0033040235021,-13.6239537563916,51.4944004709448));
#3072=CARTESIAN_POINT('Ctrl Pts',(53.1286205132889,-12.8983806298848,51.8853576341468));
#3073=CARTESIAN_POINT('Ctrl Pts',(51.1333216249648,-13.1430309825168,52.2763147973489));
#3074=CARTESIAN_POINT('Ctrl Pts',(49.4894537168485,-14.3000624425198,52.6672719605509));
#3075=CARTESIAN_POINT('Ctrl Pts',(48.5858529064304,-16.0957627348048,53.058229123753));
#3076=CARTESIAN_POINT('Ctrl Pts',(48.6362782841291,-18.1053635807713,53.449186286955));
#3077=CARTESIAN_POINT('Ctrl Pts',(49.6287966382981,-19.8534884080997,53.840143450157));
#3078=CARTESIAN_POINT('Ctrl Pts',(51.3286289756928,-20.9266177184319,54.2311006133591));
#3079=CARTESIAN_POINT('Ctrl Pts',(53.3336769082637,-21.0709008598302,54.6220577765612));
#3080=CARTESIAN_POINT('Ctrl Pts',(55.1696445359752,-20.2522077992154,55.0130149397632));
#3081=CARTESIAN_POINT('Ctrl Pts',(56.402231363278,-18.6642011818098,55.4039721029652));
#3082=CARTESIAN_POINT('Ctrl Pts',(56.7398676601745,-16.6825258736536,55.7949292661673));
#3083=CARTESIAN_POINT('Ctrl Pts',(56.1026851208883,-14.7759494270608,56.1858864293693));
#3084=CARTESIAN_POINT('Ctrl Pts',(54.6414100340784,-13.3954747168676,56.5768435925714));
#3085=CARTESIAN_POINT('Ctrl Pts',(52.701708698725,-12.8676546237047,56.9678007557734));
#3086=CARTESIAN_POINT('Ctrl Pts',(50.7424197110664,-13.3173456033045,57.3587579189754));
#3087=CARTESIAN_POINT('Ctrl Pts',(49.2270151419221,-14.6381727336246,57.7497150821775));
#3088=CARTESIAN_POINT('Ctrl Pts',(48.5139656935336,-16.5176928320245,58.1406722453795));
#3089=CARTESIAN_POINT('Ctrl Pts',(48.7719440360339,-18.5113032479999,58.5316294085816));
#3090=CARTESIAN_POINT('Ctrl Pts',(49.9399250947533,-20.1474131350837,58.9225865717836));
#3091=CARTESIAN_POINT('Ctrl Pts',(51.7416216010786,-21.0389988096439,59.3135437349857));
#3092=CARTESIAN_POINT('Ctrl Pts',(53.7508401654488,-20.9751546505726,59.7045008981877));
#3093=CARTESIAN_POINT('Ctrl Pts',(55.4922978157049,-19.9709830674272,60.0954580613898));
#3094=CARTESIAN_POINT('Ctrl Pts',(56.5540507332295,-18.264022008069,60.4864152245918));
#3095=CARTESIAN_POINT('Ctrl Pts',(56.6849400390068,-16.2580550827007,60.8773723877939));
#3096=CARTESIAN_POINT('Ctrl Pts',(55.8540037165742,-14.4275960844986,61.2683295509959));
#3097=CARTESIAN_POINT('Ctrl Pts',(54.2578007127701,-13.2056422037469,61.659286714198));
#3098=CARTESIAN_POINT('Ctrl Pts',(52.2739146918285,-12.8812480423474,62.0502438774));
#3099=CARTESIAN_POINT('Ctrl Pts',(50.371636183478,-13.5311494138686,62.4412010406021));
#3100=CARTESIAN_POINT('Ctrl Pts',(49.0009513660834,-15.0016113982127,62.832158203804));
#3101=CARTESIAN_POINT('Ctrl Pts',(48.4860973164001,-16.9447945145355,63.2231153670061));
#3102=CARTESIAN_POINT('Ctrl Pts',(48.9488633545595,-18.9010365522097,63.6140725302082));
#3103=CARTESIAN_POINT('Ctrl Pts',(50.2797816397201,-20.4075861976786,64.0050296934103));
#3104=CARTESIAN_POINT('Ctrl Pts',(52.1640219142586,-21.1080673921761,64.3959868566123));
#3105=CARTESIAN_POINT('Ctrl Pts',(54.1558649648531,-20.8367805000576,64.7869440198143));
#3106=CARTESIAN_POINT('Ctrl Pts',(55.7841380172204,-19.6578987490017,65.1779011830163));
#3107=CARTESIAN_POINT('Ctrl Pts',(56.6636712000959,-17.8502879788808,65.5688583462184));
#3108=CARTESIAN_POINT('Ctrl Pts',(56.5864099231727,-15.8415406052356,65.9598155094205));
#3109=CARTESIAN_POINT('Ctrl Pts',(55.5706304307445,-14.1068281394938,66.3507726726225));
#3110=CARTESIAN_POINT('Ctrl Pts',(53.8566165350199,-13.0564988190924,66.7417298358246));
#3111=CARTESIAN_POINT('Ctrl Pts',(51.8498202027826,-12.9390092579546,67.1326869990265));
#3112=CARTESIAN_POINT('Ctrl Pts',(50.0249514243833,-13.7821517474598,67.5236441622287));
#3113=CARTESIAN_POINT('Ctrl Pts',(48.8136850171062,-15.3864799578778,67.9146013254307));
#3114=CARTESIAN_POINT('Ctrl Pts',(48.5025474487642,-17.3724881979037,68.3055584886327));
#3115=CARTESIAN_POINT('Ctrl Pts',(49.1651386702972,-19.2703839245662,68.6965156518348));
#3116=CARTESIAN_POINT('Ctrl Pts',(50.6447219634242,-20.6312177112838,69.0874728150368));
#3117=CARTESIAN_POINT('Ctrl Pts',(52.5913001901039,-21.1330827546075,69.4784299782389));
#3118=CARTESIAN_POINT('Ctrl Pts',(54.5444080247444,-20.657262297519,69.8693871414409));
#3119=CARTESIAN_POINT('Ctrl Pts',(56.0420355481367,-19.3163122216428,70.2603443046429));
#3120=CARTESIAN_POINT('Ctrl Pts',(56.72991725061,-17.427435809996,70.651301467845));
#3121=CARTESIAN_POINT('Ctrl Pts',(56.4453338975223,-15.4374489730838,71.042258631047));
#3122=CARTESIAN_POINT('Ctrl Pts',(55.255604060317,-13.8170853662882,71.4332157942491));
#3123=CARTESIAN_POINT('Ctrl Pts',(53.4421595967455,-12.9496439359626,71.8241729574512));
#3124=CARTESIAN_POINT('Ctrl Pts',(51.4339731256248,-13.0403188167553,72.2151301206532));
#3125=CARTESIAN_POINT('Ctrl Pts',(49.7060829637914,-14.067661057971,72.6060872838552));
#3126=CARTESIAN_POINT('Ctrl Pts',(48.6672246276916,-15.7886510209866,72.9970444470573));
#3127=CARTESIAN_POINT('Ctrl Pts',(48.5631388489693,-17.7961879271213,73.3880016102593));
#3128=CARTESIAN_POINT('Ctrl Pts',(49.4184523520201,-19.6153835669027,73.7789587734614));
#3129=CARTESIAN_POINT('Ctrl Pts',(51.0308282898254,-20.8159115065848,74.1699159366634));
#3130=CARTESIAN_POINT('Ctrl Pts',(53.0188804033209,-21.1137709412463,74.5608730998655));
#3131=CARTESIAN_POINT('Ctrl Pts',(54.912275787121,-20.4385313200904,74.9518302630675));
#3132=CARTESIAN_POINT('Ctrl Pts',(56.2632251605407,-18.9498488446407,75.3427874262696));
#3133=CARTESIAN_POINT('Ctrl Pts',(56.5889499519861,-17.6499166343259,75.6034255350709));
#3134=CARTESIAN_POINT('Ctrl Pts',(56.5889499519861,-17.,75.7337445894716));
#3135=CARTESIAN_POINT('Ctrl Pts',(57.3618632631907,-17.1267342853886,51.3345782519786));
#3136=CARTESIAN_POINT('Ctrl Pts',(57.3826228523727,-16.3498182766226,51.4648973063793));
#3137=CARTESIAN_POINT('Ctrl Pts',(57.0352479861203,-14.7868998097433,51.7255354151806));
#3138=CARTESIAN_POINT('Ctrl Pts',(55.4686698444437,-12.9648823336634,52.1164925783827));
#3139=CARTESIAN_POINT('Ctrl Pts',(53.2281208840586,-12.0978291083762,52.5074497415848));
#3140=CARTESIAN_POINT('Ctrl Pts',(50.8433451463302,-12.3901715913768,52.8984069047868));
#3141=CARTESIAN_POINT('Ctrl Pts',(48.8786212540224,-13.7730726787602,53.2893640679889));
#3142=CARTESIAN_POINT('Ctrl Pts',(47.7986434171988,-15.9192610497727,53.6803212311909));
#3143=CARTESIAN_POINT('Ctrl Pts',(47.8589131842379,-18.3211206357986,54.0712783943929));
#3144=CARTESIAN_POINT('Ctrl Pts',(49.0451596110562,-20.4104577860508,54.462235557595));
#3145=CARTESIAN_POINT('Ctrl Pts',(51.0767813625441,-21.6930517414687,54.853192720797));
#3146=CARTESIAN_POINT('Ctrl Pts',(53.4731929325189,-21.8654967884011,55.2441498839991));
#3147=CARTESIAN_POINT('Ctrl Pts',(55.6675218063666,-20.8870039199405,55.6351070472011));
#3148=CARTESIAN_POINT('Ctrl Pts',(57.1406963040962,-18.9890353360354,56.0260642104031));
#3149=CARTESIAN_POINT('Ctrl Pts',(57.5442355978115,-16.6205583533319,56.4170213736052));
#3150=CARTESIAN_POINT('Ctrl Pts',(56.782681862343,-14.3418386345305,56.8079785368072));
#3151=CARTESIAN_POINT('Ctrl Pts',(55.0361815778019,-12.6919101013593,57.1989357000093));
#3152=CARTESIAN_POINT('Ctrl Pts',(52.7178713740276,-12.0610651892422,57.5898928632113));
#3153=CARTESIAN_POINT('Ctrl Pts',(50.3761502212309,-12.598531020774,57.9808500264134));
#3154=CARTESIAN_POINT('Ctrl Pts',(48.5649549565342,-14.1771694188471,58.3718071896154));
#3155=CARTESIAN_POINT('Ctrl Pts',(47.7127259147526,-16.4235516534108,58.7627643528175));
#3156=CARTESIAN_POINT('Ctrl Pts',(48.021058858721,-18.8062934092461,59.1537215160195));
#3157=CARTESIAN_POINT('Ctrl Pts',(49.4170172750347,-20.7617543732099,59.5446786792216));
#3158=CARTESIAN_POINT('Ctrl Pts',(51.5703855876311,-21.8273679950004,59.9356358424236));
#3159=CARTESIAN_POINT('Ctrl Pts',(53.9717820350656,-21.7510621418458,60.3265930056256));
#3160=CARTESIAN_POINT('Ctrl Pts',(56.0531535139181,-20.550887051311,60.7175501688278));
#3161=CARTESIAN_POINT('Ctrl Pts',(57.3221491968199,-18.5107455273791,61.1085073320297));
#3162=CARTESIAN_POINT('Ctrl Pts',(57.4785866892221,-16.1132354039597,61.4994644952318));
#3163=CARTESIAN_POINT('Ctrl Pts',(56.4854605216108,-13.9254904699895,61.8904216584338));
#3164=CARTESIAN_POINT('Ctrl Pts',(54.5776958360358,-12.4650243165339,62.2813788216359));
#3165=CARTESIAN_POINT('Ctrl Pts',(52.2065765724224,-12.0773118990975,62.6723359848379));
#3166=CARTESIAN_POINT('Ctrl Pts',(49.9329937313239,-12.8540670378484,63.06329314804));
#3167=CARTESIAN_POINT('Ctrl Pts',(48.2947659598895,-14.6115474075297,63.454250311242));
#3168=CARTESIAN_POINT('Ctrl Pts',(47.6794179296765,-16.9340189967265,63.8452074744441));
#3169=CARTESIAN_POINT('Ctrl Pts',(48.2325109279855,-19.2720984684587,64.2361646376461));
#3170=CARTESIAN_POINT('Ctrl Pts',(49.82321016722,-21.0727104231042,64.6271218008482));
#3171=CARTESIAN_POINT('Ctrl Pts',(52.0752339050124,-21.9099180230063,65.0180789640502));
#3172=CARTESIAN_POINT('Ctrl Pts',(54.4558633250017,-21.5856788433975,65.4090361272523));
#3173=CARTESIAN_POINT('Ctrl Pts',(56.4019577881599,-20.1766920367232,65.7999932904543));
#3174=CARTESIAN_POINT('Ctrl Pts',(57.4531664014012,-18.0162550595463,66.1909504536564));
#3175=CARTESIAN_POINT('Ctrl Pts',(57.3608245530749,-15.6154217742106,66.5819076168584));
#3176=CARTESIAN_POINT('Ctrl Pts',(56.1467758140548,-13.5421120674427,66.9728647800605));
#3177=CARTESIAN_POINT('Ctrl Pts',(54.0982048158494,-12.2867697451128,67.3638219432625));
#3178=CARTESIAN_POINT('Ctrl Pts',(51.6997033942426,-12.1463474836051,67.7547791064645));
#3179=CARTESIAN_POINT('Ctrl Pts',(49.5186398309548,-13.1540623309393,68.1457362696666));
#3180=CARTESIAN_POINT('Ctrl Pts',(48.0709472309629,-15.0715381763131,68.5366934328686));
#3181=CARTESIAN_POINT('Ctrl Pts',(47.6990789512508,-17.4451938931097,68.9276505960707));
#3182=CARTESIAN_POINT('Ctrl Pts',(48.491000862243,-19.7135384811981,69.3186077592727));
#3183=CARTESIAN_POINT('Ctrl Pts',(50.2593829226289,-21.3399924053029,69.7095649224748));
#3184=CARTESIAN_POINT('Ctrl Pts',(52.585912310354,-21.9398161173807,70.1005220856768));
#3185=CARTESIAN_POINT('Ctrl Pts',(54.9202458182389,-21.3711206118296,70.4914792488789));
#3186=CARTESIAN_POINT('Ctrl Pts',(56.7101941441817,-19.7684314969577,70.8824364120809));
#3187=CARTESIAN_POINT('Ctrl Pts',(57.5323429756866,-17.5108666700446,71.273393575283));
#3188=CARTESIAN_POINT('Ctrl Pts',(57.1922119889622,-15.1324558369381,71.664350738485));
#3189=CARTESIAN_POINT('Ctrl Pts',(55.7702597089705,-13.1958145279503,72.055307901687));
#3190=CARTESIAN_POINT('Ctrl Pts',(53.602850271426,-12.159058129237,72.4462650648891));
#3191=CARTESIAN_POINT('Ctrl Pts',(51.2026875702207,-12.267431164002,72.8372222280911));
#3192=CARTESIAN_POINT('Ctrl Pts',(49.1375313729449,-13.495300895059,73.2281793912932));
#3193=CARTESIAN_POINT('Ctrl Pts',(47.8958999737314,-15.5522067706523,73.6191365544952));
#3194=CARTESIAN_POINT('Ctrl Pts',(47.7714957057545,-17.9515995050567,74.0100937176972));
#3195=CARTESIAN_POINT('Ctrl Pts',(48.7937614261677,-20.1258693707283,74.4010508808993));
#3196=CARTESIAN_POINT('Ctrl Pts',(50.7208456688109,-21.5607567224907,74.7920080441013));
#3197=CARTESIAN_POINT('Ctrl Pts',(53.0969617625352,-21.9166945762927,75.1829652073034));
#3198=CARTESIAN_POINT('Ctrl Pts',(55.3598711261245,-21.1097979586625,75.5739223705055));
#3199=CARTESIAN_POINT('Ctrl Pts',(56.974558168743,-19.3302754071,75.9648795337075));
#3200=CARTESIAN_POINT('Ctrl Pts',(57.3635561632098,-17.7771933126448,76.2255176425089));
#3201=CARTESIAN_POINT('Ctrl Pts',(57.3635561632098,-17.,76.3558366969096));
#3202=CARTESIAN_POINT('Ctrl Pts',(58.3303540870803,-17.1526128506436,51.1101091552529));
#3203=CARTESIAN_POINT('Ctrl Pts',(58.355341642541,-16.2174675697245,51.2404282096536));
#3204=CARTESIAN_POINT('Ctrl Pts',(57.9367994837362,-14.3349762708849,51.5010663184549));
#3205=CARTESIAN_POINT('Ctrl Pts',(56.0504566417972,-12.1412485071656,51.8920234816569));
#3206=CARTESIAN_POINT('Ctrl Pts',(53.3524778992612,-11.097069130456,52.282980644859));
#3207=CARTESIAN_POINT('Ctrl Pts',(50.480890442206,-11.4491438159843,52.6739378080611));
#3208=CARTESIAN_POINT('Ctrl Pts',(48.1150815112142,-13.1143229732784,53.0648949712631));
#3209=CARTESIAN_POINT('Ctrl Pts',(46.8146414639397,-15.6986438445251,53.4558521344651));
#3210=CARTESIAN_POINT('Ctrl Pts',(46.8872129710008,-18.5908111680355,53.8468092976672));
#3211=CARTESIAN_POINT('Ctrl Pts',(48.3156193136198,-21.1066660539386,54.2377664608693));
#3212=CARTESIAN_POINT('Ctrl Pts',(50.7619739606184,-22.6510862949705,54.6287236240713));
#3213=CARTESIAN_POINT('Ctrl Pts',(53.6475867703978,-22.8587346431059,55.0196807872733));
#3214=CARTESIAN_POINT('Ctrl Pts',(56.2898636869932,-21.680492961833,55.4106379504754));
#3215=CARTESIAN_POINT('Ctrl Pts',(58.0637705985691,-19.3950750712552,55.8015951136774));
#3216=CARTESIAN_POINT('Ctrl Pts',(58.5496879870503,-16.5430994954114,56.1925522768795));
#3217=CARTESIAN_POINT('Ctrl Pts',(57.6326714355344,-13.7992042203998,56.5835094400815));
#3218=CARTESIAN_POINT('Ctrl Pts',(55.5296423135302,-11.8124609031937,56.9744666032836));
#3219=CARTESIAN_POINT('Ctrl Pts',(52.7380745681098,-11.0528359423474,57.3654237664856));
#3220=CARTESIAN_POINT('Ctrl Pts',(49.9183167834665,-11.7000195126523,57.7563809296876));
#3221=CARTESIAN_POINT('Ctrl Pts',(47.7373859160472,-13.6009195870612,58.1473380928897));
#3222=CARTESIAN_POINT('Ctrl Pts',(46.7111836836696,-16.305876060109,58.5382952560918));
#3223=CARTESIAN_POINT('Ctrl Pts',(47.0824594087586,-19.1750283524781,58.9292524192938));
#3224=CARTESIAN_POINT('Ctrl Pts',(48.7633873901451,-21.5296751760025,59.3202095824958));
#3225=CARTESIAN_POINT('Ctrl Pts',(51.3563421720835,-22.812822104585,59.7111667456979));
#3226=CARTESIAN_POINT('Ctrl Pts',(54.2479573060245,-22.7209392503051,60.1021239088999));
#3227=CARTESIAN_POINT('Ctrl Pts',(56.7542178920496,-21.275761608413,60.493081072102));
#3228=CARTESIAN_POINT('Ctrl Pts',(58.2822650937144,-18.8191476193684,60.884038235304));
#3229=CARTESIAN_POINT('Ctrl Pts',(58.4706375804947,-15.9322121597635,61.2749953985061));
#3230=CARTESIAN_POINT('Ctrl Pts',(57.2747756230685,-13.2978631471098,61.6659525617081));
#3231=CARTESIAN_POINT('Ctrl Pts',(54.9775617487357,-11.5392588831358,62.0569097249102));
#3232=CARTESIAN_POINT('Ctrl Pts',(52.1224045528526,-11.0723992377504,62.4478668881122));
#3233=CARTESIAN_POINT('Ctrl Pts',(49.3846947679361,-12.007720399312,62.8388240513143));
#3234=CARTESIAN_POINT('Ctrl Pts',(47.4120408057822,-14.1239710667169,63.2297812145162));
#3235=CARTESIAN_POINT('Ctrl Pts',(46.6710762396398,-16.9205497002286,63.6207383777184));
#3236=CARTESIAN_POINT('Ctrl Pts',(47.3370770934763,-19.7359223939198,64.0116955409204));
#3237=CARTESIAN_POINT('Ctrl Pts',(49.2525000960564,-21.9041094852197,64.4026527041224));
#3238=CARTESIAN_POINT('Ctrl Pts',(51.9642497237231,-22.9122238133307,64.7936098673245));
#3239=CARTESIAN_POINT('Ctrl Pts',(54.8308584698625,-22.5217947695224,65.1845670305265));
#3240=CARTESIAN_POINT('Ctrl Pts',(57.1742267245179,-20.8251787950697,65.5755241937285));
#3241=CARTESIAN_POINT('Ctrl Pts',(58.4400280203571,-18.2237123583959,65.9664813569306));
#3242=CARTESIAN_POINT('Ctrl Pts',(58.3288355987958,-15.3327753499006,66.3574385201327));
#3243=CARTESIAN_POINT('Ctrl Pts',(56.8669521555819,-12.8362222581074,66.7483956833347));
#3244=CARTESIAN_POINT('Ctrl Pts',(54.4001879077564,-11.3246156004952,67.1393528465368));
#3245=CARTESIAN_POINT('Ctrl Pts',(51.5120587873418,-11.1555276779201,67.5303100097388));
#3246=CARTESIAN_POINT('Ctrl Pts',(48.8857550737321,-12.3689564337142,67.9212671729409));
#3247=CARTESIAN_POINT('Ctrl Pts',(47.1425319437795,-14.6778638942547,68.3122243361429));
#3248=CARTESIAN_POINT('Ctrl Pts',(46.6947508425837,-17.536075332595,68.7031814993449));
#3249=CARTESIAN_POINT('Ctrl Pts',(47.6483349063834,-20.2674775322146,69.094138662547));
#3250=CARTESIAN_POINT('Ctrl Pts',(49.7777127244415,-22.2259541466555,69.485095825749));
#3251=CARTESIAN_POINT('Ctrl Pts',(52.5791775122401,-22.9482252733484,69.8760529889511));
#3252=CARTESIAN_POINT('Ctrl Pts',(55.3900395430226,-22.2634368371744,70.2670101521531));
#3253=CARTESIAN_POINT('Ctrl Pts',(57.5453861467663,-20.3335763463122,70.6579673153551));
#3254=CARTESIAN_POINT('Ctrl Pts',(58.5353676164029,-17.6151545016087,71.0489244785573));
#3255=CARTESIAN_POINT('Ctrl Pts',(58.1258026451683,-14.7512171894498,71.4398816417592));
#3256=CARTESIAN_POINT('Ctrl Pts',(56.4135744009266,-12.4192319611238,71.8308388049613));
#3257=CARTESIAN_POINT('Ctrl Pts',(53.8037122342891,-11.1708328924698,72.2217959681633));
#3258=CARTESIAN_POINT('Ctrl Pts',(50.9135825266937,-11.3013296269896,72.6127531313654));
#3259=CARTESIAN_POINT('Ctrl Pts',(48.4268477765921,-12.7798543046457,73.0037102945674));
#3260=CARTESIAN_POINT('Ctrl Pts',(46.9317501611453,-15.2566574068001,73.3946674577695));
#3261=CARTESIAN_POINT('Ctrl Pts',(46.7819519459475,-18.1458543446259,73.7856246209715));
#3262=CARTESIAN_POINT('Ctrl Pts',(48.0128982703705,-20.7639891441552,74.1765817841736));
#3263=CARTESIAN_POINT('Ctrl Pts',(50.3333845221266,-22.4917672199676,74.5675389473756));
#3264=CARTESIAN_POINT('Ctrl Pts',(53.1945431347214,-22.9204191781828,74.9584961105777));
#3265=CARTESIAN_POINT('Ctrl Pts',(55.9194502805027,-21.9486780023587,75.3494532737797));
#3266=CARTESIAN_POINT('Ctrl Pts',(57.8637166740634,-19.8061190161188,75.7404104369818));
#3267=CARTESIAN_POINT('Ctrl Pts',(58.3323926695916,-17.9354790614188,76.0010485457831));
#3268=CARTESIAN_POINT('Ctrl Pts',(58.3323926695916,-17.,76.1313676001838));
#3269=CARTESIAN_POINT('Ctrl Pts',(58.6167627387145,-17.1602658348517,50.515747952988));
#3270=CARTESIAN_POINT('Ctrl Pts',(58.643021929101,-16.1775303283992,50.6460670073887));
#3271=CARTESIAN_POINT('Ctrl Pts',(58.2038868966466,-14.2013661449526,50.90670511619));
#3272=CARTESIAN_POINT('Ctrl Pts',(56.2227429467729,-11.8970628069899,51.2976622793921));
#3273=CARTESIAN_POINT('Ctrl Pts',(53.3893353851998,-10.8006526176493,51.6886194425942));
#3274=CARTESIAN_POINT('Ctrl Pts',(50.3734979083497,-11.1703199580457,52.0795766057962));
#3275=CARTESIAN_POINT('Ctrl Pts',(47.8888793667432,-12.9191770184205,52.4705337689982));
#3276=CARTESIAN_POINT('Ctrl Pts',(46.5231185913547,-15.6332764679385,52.8614909322003));
#3277=CARTESIAN_POINT('Ctrl Pts',(46.5993378377957,-18.670713066158,53.2524480954023));
#3278=CARTESIAN_POINT('Ctrl Pts',(48.0994850847202,-21.3129233154427,53.6434052586044));
#3279=CARTESIAN_POINT('Ctrl Pts',(50.6687092654925,-22.9349145267153,54.0343624218064));
#3280=CARTESIAN_POINT('Ctrl Pts',(53.6992526266351,-23.1529911692309,54.4253195850084));
#3281=CARTESIAN_POINT('Ctrl Pts',(56.474238869349,-21.9155723452686,54.8162767482105));
#3282=CARTESIAN_POINT('Ctrl Pts',(58.3372407626147,-19.5153684182812,55.2072339114125));
#3283=CARTESIAN_POINT('Ctrl Pts',(58.8475635336849,-16.5201515504479,55.5981910746146));
#3284=CARTESIAN_POINT('Ctrl Pts',(57.8844895212394,-13.6384432193433,55.9891482378167));
#3285=CARTESIAN_POINT('Ctrl Pts',(55.6758350972527,-11.5519151052446,56.3801054010187));
#3286=CARTESIAN_POINT('Ctrl Pts',(52.7440599696852,-10.7541377298025,56.7710625642207));
#3287=CARTESIAN_POINT('Ctrl Pts',(49.7826789530834,-11.433826305252,57.1620197274228));
#3288=CARTESIAN_POINT('Ctrl Pts',(47.4922101373727,-13.4301996896761,57.5529768906249));
#3289=CARTESIAN_POINT('Ctrl Pts',(46.4144665711598,-16.2710134643385,57.9439340538269));
#3290=CARTESIAN_POINT('Ctrl Pts',(46.8043897377188,-19.2842698443785,58.3348912170289));
#3291=CARTESIAN_POINT('Ctrl Pts',(48.569742862618,-21.7571795550599,58.7258483802309));
#3292=CARTESIAN_POINT('Ctrl Pts',(51.2929296246423,-23.1047729468906,59.116805543433));
#3293=CARTESIAN_POINT('Ctrl Pts',(54.3297770500483,-23.0082752470182,59.507762706635));
#3294=CARTESIAN_POINT('Ctrl Pts',(56.9619153725668,-21.4905130975688,59.8987198698371));
#3295=CARTESIAN_POINT('Ctrl Pts',(58.566709231817,-18.910514888186,60.2896770330391));
#3296=CARTESIAN_POINT('Ctrl Pts',(58.7645427867655,-15.8785821752588,60.6806341962412));
#3297=CARTESIAN_POINT('Ctrl Pts',(57.5086182814925,-13.111922144068,61.0715913594432));
#3298=CARTESIAN_POINT('Ctrl Pts',(55.0960261083635,-11.2649914205938,61.4625485226453));
#3299=CARTESIAN_POINT('Ctrl Pts',(52.0974677325831,-10.7746836007645,61.8535056858473));
#3300=CARTESIAN_POINT('Ctrl Pts',(49.2222556014069,-11.7569815656853,62.2444628490494));
#3301=CARTESIAN_POINT('Ctrl Pts',(47.1505244654603,-13.9795215971582,62.6354200122514));
#3302=CARTESIAN_POINT('Ctrl Pts',(46.3723447178911,-16.9165592836075,63.0263771754535));
#3303=CARTESIAN_POINT('Ctrl Pts',(47.0717956768182,-19.873334967897,63.4173343386555));
#3304=CARTESIAN_POINT('Ctrl Pts',(49.0834214100111,-22.1504199467036,63.8082915018576));
#3305=CARTESIAN_POINT('Ctrl Pts',(51.9313695267679,-23.2091671381576,64.1992486650596));
#3306=CARTESIAN_POINT('Ctrl Pts',(54.9419546105651,-22.7991286712227,64.5902058282616));
#3307=CARTESIAN_POINT('Ctrl Pts',(57.4030192824745,-21.0172996188621,64.9811629914637));
#3308=CARTESIAN_POINT('Ctrl Pts',(58.7323958517169,-18.2851737015071,65.3721201546658));
#3309=CARTESIAN_POINT('Ctrl Pts',(58.6156187553549,-15.2490384606216,65.7630773178678));
#3310=CARTESIAN_POINT('Ctrl Pts',(57.0803117504052,-12.6270951943288,66.1540344810699));
#3311=CARTESIAN_POINT('Ctrl Pts',(54.4896534822575,-11.0395676106787,66.5449916442719));
#3312=CARTESIAN_POINT('Ctrl Pts',(51.456467156517,-10.861987193356,66.9359488074739));
#3313=CARTESIAN_POINT('Ctrl Pts',(48.6982565021046,-12.1363607949564,67.326905970676));
#3314=CARTESIAN_POINT('Ctrl Pts',(46.8674794349484,-14.5612338685727,67.717863133878));
#3315=CARTESIAN_POINT('Ctrl Pts',(46.3972083854018,-17.5629998867075,68.1088202970801));
#3316=CARTESIAN_POINT('Ctrl Pts',(47.3986865123584,-20.4315876329779,68.4997774602821));
#3317=CARTESIAN_POINT('Ctrl Pts',(49.6350130104282,-22.4884293575185,68.8907346234842));
#3318=CARTESIAN_POINT('Ctrl Pts',(52.5771822584804,-23.2469767857663,69.2816917866862));
#3319=CARTESIAN_POINT('Ctrl Pts',(55.5292207332768,-22.5277946233674,69.6726489498883));
#3320=CARTESIAN_POINT('Ctrl Pts',(57.7928203006812,-20.5010062935296,70.0636061130903));
#3321=CARTESIAN_POINT('Ctrl Pts',(58.8325239186161,-17.6460508042341,70.4545632762924));
#3322=CARTESIAN_POINT('Ctrl Pts',(58.4023883868815,-14.6382714173167,70.8455204394944));
#3323=CARTESIAN_POINT('Ctrl Pts',(56.6041629968483,-12.1891612948279,71.2364776026964));
#3324=CARTESIAN_POINT('Ctrl Pts',(53.8632195340322,-10.8780614028313,71.6274347658985));
#3325=CARTESIAN_POINT('Ctrl Pts',(50.8279324366534,-11.01511147493,72.0183919291005));
#3326=CARTESIAN_POINT('Ctrl Pts',(48.2162999967831,-12.5678974806397,72.4093490923026));
#3327=CARTESIAN_POINT('Ctrl Pts',(46.6461119996725,-15.1690945930496,72.8003062555046));
#3328=CARTESIAN_POINT('Ctrl Pts',(46.4887870630162,-18.2034115385973,73.1912634187066));
#3329=CARTESIAN_POINT('Ctrl Pts',(47.7815642969756,-20.953023391354,73.5822205819087));
#3330=CARTESIAN_POINT('Ctrl Pts',(50.2185826497119,-22.7676230340697,73.9731777451107));
#3331=CARTESIAN_POINT('Ctrl Pts',(53.2234698965323,-23.2177144283724,74.3641349083128));
#3332=CARTESIAN_POINT('Ctrl Pts',(56.0851526759193,-22.1973785114167,74.7550920715148));
#3333=CARTESIAN_POINT('Ctrl Pts',(58.1271399333403,-19.9468156342685,75.1460492347169));
#3334=CARTESIAN_POINT('Ctrl Pts',(58.6189035487885,-17.9830862732854,75.4066873435182));
#3335=CARTESIAN_POINT('Ctrl Pts',(58.6189035487885,-17.,75.5370063979189));
#3336=CARTESIAN_POINT('Ctrl Pts',(58.6167627387145,-17.1602658348517,50.2165486526461));
#3337=CARTESIAN_POINT('Ctrl Pts',(58.643008473399,-16.178033900518,50.3468677070468));
#3338=CARTESIAN_POINT('Ctrl Pts',(58.2035873080419,-14.2013435692345,50.6075058158482));
#3339=CARTESIAN_POINT('Ctrl Pts',(56.2225937043736,-11.897451182557,50.9984629790502));
#3340=CARTESIAN_POINT('Ctrl Pts',(53.3892837467024,-10.8009462068176,51.3894201422522));
#3341=CARTESIAN_POINT('Ctrl Pts',(50.3736273245558,-11.1706588511001,51.7803773054543));
#3342=CARTESIAN_POINT('Ctrl Pts',(47.8891338131767,-12.9193891815025,52.1713344686563));
#3343=CARTESIAN_POINT('Ctrl Pts',(46.523451423545,-15.6333553665913,52.5622916318584));
#3344=CARTESIAN_POINT('Ctrl Pts',(46.599664491672,-18.6706201350726,52.9532487950604));
#3345=CARTESIAN_POINT('Ctrl Pts',(48.0997310899548,-21.3126898076219,53.3442059582625));
#3346=CARTESIAN_POINT('Ctrl Pts',(50.66881515933,-22.9345914086011,53.7351631214646));
#3347=CARTESIAN_POINT('Ctrl Pts',(53.6991939529023,-23.1526568531196,54.1261202846665));
#3348=CARTESIAN_POINT('Ctrl Pts',(56.47402923455,-21.9153050002011,54.5170774478686));
#3349=CARTESIAN_POINT('Ctrl Pts',(58.3369298825998,-19.5152317078047,54.9080346110706));
#3350=CARTESIAN_POINT('Ctrl Pts',(58.8472248890723,-16.5201776181574,55.2989917742727));
#3351=CARTESIAN_POINT('Ctrl Pts',(57.8842032458303,-13.6386259892673,55.6899489374747));
#3352=CARTESIAN_POINT('Ctrl Pts',(55.6756688973336,-11.5522113011612,56.0809061006768));
#3353=CARTESIAN_POINT('Ctrl Pts',(52.7440531658162,-10.7544773055472,56.4718632638789));
#3354=CARTESIAN_POINT('Ctrl Pts',(49.7828331520566,-11.4341289248563,56.8628204270809));
#3355=CARTESIAN_POINT('Ctrl Pts',(47.4924888644779,-13.430393772254,57.253777590283));
#3356=CARTESIAN_POINT('Ctrl Pts',(46.4148038926073,-16.271053097522,57.644734753485));
#3357=CARTESIAN_POINT('Ctrl Pts',(46.8047058599946,-19.2841456537754,58.035691916687));
#3358=CARTESIAN_POINT('Ctrl Pts',(48.5699630065106,-21.7569209176924,58.4266490798891));
#3359=CARTESIAN_POINT('Ctrl Pts',(51.293001714916,-23.1044410439156,58.8176062430911));
#3360=CARTESIAN_POINT('Ctrl Pts',(54.3296840336396,-23.0079485903805,59.2085634062931));
#3361=CARTESIAN_POINT('Ctrl Pts',(56.9616792526266,-21.4902689583137,59.5995205694953));
#3362=CARTESIAN_POINT('Ctrl Pts',(58.5663858627843,-18.9104110177176,59.9904777326972));
#3363=CARTESIAN_POINT('Ctrl Pts',(58.7642086619611,-15.8786431442651,60.3814348958993));
#3364=CARTESIAN_POINT('Ctrl Pts',(57.5083524385236,-13.112133530256,60.7723920591013));
#3365=CARTESIAN_POINT('Ctrl Pts',(55.095891432692,-11.2653032203185,61.1633492223034));
#3366=CARTESIAN_POINT('Ctrl Pts',(52.0974960818944,-10.77502205744,61.5543063855054));
#3367=CARTESIAN_POINT('Ctrl Pts',(49.2224402696388,-11.7572666169945,61.9452635487075));
#3368=CARTESIAN_POINT('Ctrl Pts',(47.1508217691292,-13.9796858138845,62.3362207119095));
#3369=CARTESIAN_POINT('Ctrl Pts',(46.3726843294707,-16.9165638200946,62.7271778751116));
#3370=CARTESIAN_POINT('Ctrl Pts',(47.0720972607971,-19.8731787510337,63.1181350383136));
#3371=CARTESIAN_POINT('Ctrl Pts',(49.0836136263508,-22.1501399297692,63.5090922015157));
#3372=CARTESIAN_POINT('Ctrl Pts',(51.9314069064712,-23.2088295594817,63.9000493647177));
#3373=CARTESIAN_POINT('Ctrl Pts',(54.9418283114199,-22.7988133854305,64.2910065279198));
#3374=CARTESIAN_POINT('Ctrl Pts',(57.4027591806895,-21.0170812071728,64.6819636911218));
#3375=CARTESIAN_POINT('Ctrl Pts',(58.7320634746702,-18.2851038294562,65.0729208543239));
#3376=CARTESIAN_POINT('Ctrl Pts',(58.6152927272196,-15.2491336565274,65.4638780175259));
#3377=CARTESIAN_POINT('Ctrl Pts',(57.080069193516,-12.6273329394813,65.854835180728));
#3378=CARTESIAN_POINT('Ctrl Pts',(54.4895517737208,-11.039891666206,66.24579234393));
#3379=CARTESIAN_POINT('Ctrl Pts',(51.4565303556175,-10.8623209035087,66.636749507132));
#3380=CARTESIAN_POINT('Ctrl Pts',(48.6984696589939,-12.1366252202991,67.0277066703341));
#3381=CARTESIAN_POINT('Ctrl Pts',(46.8677921271795,-14.5613664587978,67.4186638335361));
#3382=CARTESIAN_POINT('Ctrl Pts',(46.3975466451333,-17.5629692778492,67.8096209967382));
#3383=CARTESIAN_POINT('Ctrl Pts',(47.3989703241477,-20.431401064721,68.2005781599402));
#3384=CARTESIAN_POINT('Ctrl Pts',(49.6351752376468,-22.4881309646939,68.5915353231423));
#3385=CARTESIAN_POINT('Ctrl Pts',(52.5771845274374,-23.2466371494448,68.9824924863443));
#3386=CARTESIAN_POINT('Ctrl Pts',(55.529062504339,-22.5274940937726,69.3734496495464));
#3387=CARTESIAN_POINT('Ctrl Pts',(57.7925390093781,-20.5008159421237,69.7644068127484));
#3388=CARTESIAN_POINT('Ctrl Pts',(58.8321860911263,-17.6460157002987,70.1553639759505));
#3389=CARTESIAN_POINT('Ctrl Pts',(58.4020739661194,-14.6383997751071,70.5463211391525));
#3390=CARTESIAN_POINT('Ctrl Pts',(56.6039462958005,-12.189422944957,70.9372783023545));
#3391=CARTESIAN_POINT('Ctrl Pts',(53.8631519513258,-10.8783940324256,71.3282354655566));
#3392=CARTESIAN_POINT('Ctrl Pts',(50.8280296619087,-11.0154373062825,71.7191926287586));
#3393=CARTESIAN_POINT('Ctrl Pts',(48.2165396770217,-12.5681374761835,72.1101497919607));
#3394=CARTESIAN_POINT('Ctrl Pts',(46.6464360547185,-15.1691962162198,72.5011069551627));
#3395=CARTESIAN_POINT('Ctrl Pts',(46.4891218839111,-18.2033415583671,72.8920641183648));
#3396=CARTESIAN_POINT('Ctrl Pts',(47.7818243197045,-20.9528181004838,73.2830212815669));
#3397=CARTESIAN_POINT('Ctrl Pts',(50.2187210719051,-22.7672877187656,73.6739784447688));
#3398=CARTESIAN_POINT('Ctrl Pts',(53.2234261185118,-23.2174195646428,74.0649356079709));
#3399=CARTESIAN_POINT('Ctrl Pts',(56.085013860659,-22.196986288013,74.4558927711729));
#3400=CARTESIAN_POINT('Ctrl Pts',(58.1268398486099,-19.9468301996286,74.846849934375));
#3401=CARTESIAN_POINT('Ctrl Pts',(58.6189035487885,-17.9825825214271,75.1074880431764));
#3402=CARTESIAN_POINT('Ctrl Pts',(58.6189035487885,-17.,75.237807097577));
#3403=CARTESIAN_POINT('Ctrl Pts',(58.6189035487885,-17.,50.2378070975771));
#3404=CARTESIAN_POINT('Ctrl Pts',(58.6189035487885,-17.0075706036887,50.2948881046132));
#3405=CARTESIAN_POINT('Ctrl Pts',(58.613828368086,-17.0151298524557,50.3518834975562));
#3406=CARTESIAN_POINT('Ctrl Pts',(58.591050565214,-17.0319486181224,50.4786940031426));
#3407=CARTESIAN_POINT('Ctrl Pts',(58.5705467068289,-17.0410922984269,50.5476357284341));
#3408=CARTESIAN_POINT('Ctrl Pts',(58.5425991292395,-17.0498583740029,50.6137303811466));
#3409=CARTESIAN_POINT('Ctrl Pts',(58.4930513356688,-17.0653996029939,50.7309084871288));
#3410=CARTESIAN_POINT('Ctrl Pts',(58.4208808497062,-17.0795128662973,50.8373199854651));
#3411=CARTESIAN_POINT('Ctrl Pts',(58.238833135979,-17.1034494723391,51.0177977431282));
#3412=CARTESIAN_POINT('Ctrl Pts',(58.1304335946722,-17.1130008760904,51.0898136307712));
#3413=CARTESIAN_POINT('Ctrl Pts',(57.8907803690335,-17.1262287645946,51.1895495604053));
#3414=CARTESIAN_POINT('Ctrl Pts',(57.7615831682544,-17.129718953074,51.2158649615548));
#3415=CARTESIAN_POINT('Ctrl Pts',(57.4993934087917,-17.1300465850083,51.2183352481413));
#3416=CARTESIAN_POINT('Ctrl Pts',(57.368745871217,-17.1268329794921,51.1941052333931));
#3417=CARTESIAN_POINT('Ctrl Pts',(57.1245157234726,-17.1140335739622,51.0975999892737));
#3418=CARTESIAN_POINT('Ctrl Pts',(57.0130468177773,-17.1045699914424,51.0262462581385));
#3419=CARTESIAN_POINT('Ctrl Pts',(56.8256541159993,-17.0806911803295,50.8462042639738));
#3420=CARTESIAN_POINT('Ctrl Pts',(56.7510105620165,-17.0665594245304,50.7396533355259));
#3421=CARTESIAN_POINT('Ctrl Pts',(56.6487475381862,-17.0355622762965,50.5059403439088));
#3422=CARTESIAN_POINT('Ctrl Pts',(56.6213788689869,-17.0190611114582,50.3815244925668));
#3423=CARTESIAN_POINT('Ctrl Pts',(56.6189569176101,-17.0015451233,50.2494570532432));
#3424=CARTESIAN_POINT('Ctrl Pts',(56.6189035487885,-17.0007723877109,50.2436307637169));
#3425=CARTESIAN_POINT('Ctrl Pts',(56.6189035487885,-17.,50.2378070975769));
#3426=CARTESIAN_POINT('',(58.6189035487885,-17.,75.237807097577));
#3427=CARTESIAN_POINT('Ctrl Pts',(58.6188665834176,-17.0000025997527,50.237807097577));
#3428=CARTESIAN_POINT('Ctrl Pts',(58.6184633923052,-16.0708764078228,50.3610400036674));
#3429=CARTESIAN_POINT('Ctrl Pts',(58.1676815470056,-14.1595852266855,50.6145919641585));
#3430=CARTESIAN_POINT('Ctrl Pts',(56.2225937043736,-11.897451182557,50.9984629790502));
#3431=CARTESIAN_POINT('Ctrl Pts',(53.3892837467024,-10.8009462068176,51.3894201422522));
#3432=CARTESIAN_POINT('Ctrl Pts',(50.3736273245558,-11.1706588511001,51.7803773054543));
#3433=CARTESIAN_POINT('Ctrl Pts',(47.8891338131767,-12.9193891815025,52.1713344686563));
#3434=CARTESIAN_POINT('Ctrl Pts',(46.523451423545,-15.6333553665913,52.5622916318584));
#3435=CARTESIAN_POINT('Ctrl Pts',(46.599664491672,-18.6706201350726,52.9532487950604));
#3436=CARTESIAN_POINT('Ctrl Pts',(48.0997310899548,-21.3126898076219,53.3442059582625));
#3437=CARTESIAN_POINT('Ctrl Pts',(50.66881515933,-22.9345914086011,53.7351631214646));
#3438=CARTESIAN_POINT('Ctrl Pts',(53.6991939529023,-23.1526568531196,54.1261202846665));
#3439=CARTESIAN_POINT('Ctrl Pts',(56.47402923455,-21.9153050002011,54.5170774478686));
#3440=CARTESIAN_POINT('Ctrl Pts',(58.3369298825998,-19.5152317078047,54.9080346110706));
#3441=CARTESIAN_POINT('Ctrl Pts',(58.8472248890723,-16.5201776181574,55.2989917742727));
#3442=CARTESIAN_POINT('Ctrl Pts',(57.8842032458303,-13.6386259892673,55.6899489374747));
#3443=CARTESIAN_POINT('Ctrl Pts',(55.6756688973336,-11.5522113011612,56.0809061006768));
#3444=CARTESIAN_POINT('Ctrl Pts',(52.7440531658162,-10.7544773055472,56.4718632638789));
#3445=CARTESIAN_POINT('Ctrl Pts',(49.7828331520566,-11.4341289248563,56.8628204270809));
#3446=CARTESIAN_POINT('Ctrl Pts',(47.4924888644779,-13.430393772254,57.253777590283));
#3447=CARTESIAN_POINT('Ctrl Pts',(46.4148038926073,-16.271053097522,57.644734753485));
#3448=CARTESIAN_POINT('Ctrl Pts',(46.8047058599946,-19.2841456537754,58.035691916687));
#3449=CARTESIAN_POINT('Ctrl Pts',(48.5699630065106,-21.7569209176924,58.4266490798891));
#3450=CARTESIAN_POINT('Ctrl Pts',(51.293001714916,-23.1044410439156,58.8176062430911));
#3451=CARTESIAN_POINT('Ctrl Pts',(54.3296840336396,-23.0079485903805,59.2085634062931));
#3452=CARTESIAN_POINT('Ctrl Pts',(56.9616792526266,-21.4902689583137,59.5995205694953));
#3453=CARTESIAN_POINT('Ctrl Pts',(58.5663858627843,-18.9104110177176,59.9904777326972));
#3454=CARTESIAN_POINT('Ctrl Pts',(58.7642086619611,-15.8786431442651,60.3814348958993));
#3455=CARTESIAN_POINT('Ctrl Pts',(57.5083524385236,-13.112133530256,60.7723920591013));
#3456=CARTESIAN_POINT('Ctrl Pts',(55.095891432692,-11.2653032203185,61.1633492223034));
#3457=CARTESIAN_POINT('Ctrl Pts',(52.0974960818944,-10.77502205744,61.5543063855054));
#3458=CARTESIAN_POINT('Ctrl Pts',(49.2224402696388,-11.7572666169945,61.9452635487075));
#3459=CARTESIAN_POINT('Ctrl Pts',(47.1508217691292,-13.9796858138845,62.3362207119095));
#3460=CARTESIAN_POINT('Ctrl Pts',(46.3726843294707,-16.9165638200946,62.7271778751116));
#3461=CARTESIAN_POINT('Ctrl Pts',(47.0720972607971,-19.8731787510337,63.1181350383136));
#3462=CARTESIAN_POINT('Ctrl Pts',(49.0836136263508,-22.1501399297692,63.5090922015157));
#3463=CARTESIAN_POINT('Ctrl Pts',(51.9314069064712,-23.2088295594817,63.9000493647177));
#3464=CARTESIAN_POINT('Ctrl Pts',(54.9418283114199,-22.7988133854305,64.2910065279198));
#3465=CARTESIAN_POINT('Ctrl Pts',(57.4027591806895,-21.0170812071728,64.6819636911218));
#3466=CARTESIAN_POINT('Ctrl Pts',(58.7320634746702,-18.2851038294562,65.0729208543239));
#3467=CARTESIAN_POINT('Ctrl Pts',(58.6152927272196,-15.2491336565274,65.4638780175259));
#3468=CARTESIAN_POINT('Ctrl Pts',(57.080069193516,-12.6273329394813,65.854835180728));
#3469=CARTESIAN_POINT('Ctrl Pts',(54.4895517737208,-11.039891666206,66.24579234393));
#3470=CARTESIAN_POINT('Ctrl Pts',(51.4565303556175,-10.8623209035087,66.636749507132));
#3471=CARTESIAN_POINT('Ctrl Pts',(48.6984696589939,-12.1366252202991,67.0277066703341));
#3472=CARTESIAN_POINT('Ctrl Pts',(46.8677921271795,-14.5613664587978,67.4186638335361));
#3473=CARTESIAN_POINT('Ctrl Pts',(46.3975466451333,-17.5629692778492,67.8096209967382));
#3474=CARTESIAN_POINT('Ctrl Pts',(47.3989703241477,-20.431401064721,68.2005781599402));
#3475=CARTESIAN_POINT('Ctrl Pts',(49.6351752376468,-22.4881309646939,68.5915353231423));
#3476=CARTESIAN_POINT('Ctrl Pts',(52.5771845274374,-23.2466371494448,68.9824924863443));
#3477=CARTESIAN_POINT('Ctrl Pts',(55.529062504339,-22.5274940937726,69.3734496495464));
#3478=CARTESIAN_POINT('Ctrl Pts',(57.7925390093781,-20.5008159421237,69.7644068127484));
#3479=CARTESIAN_POINT('Ctrl Pts',(58.8321860911263,-17.6460157002987,70.1553639759505));
#3480=CARTESIAN_POINT('Ctrl Pts',(58.4020739661194,-14.6383997751071,70.5463211391525));
#3481=CARTESIAN_POINT('Ctrl Pts',(56.6039462958005,-12.189422944957,70.9372783023545));
#3482=CARTESIAN_POINT('Ctrl Pts',(53.8631519513258,-10.8783940324256,71.3282354655566));
#3483=CARTESIAN_POINT('Ctrl Pts',(50.8280296619087,-11.0154373062825,71.7191926287586));
#3484=CARTESIAN_POINT('Ctrl Pts',(48.2165396770217,-12.5681374761835,72.1101497919607));
#3485=CARTESIAN_POINT('Ctrl Pts',(46.6464360547185,-15.1691962162198,72.5011069551627));
#3486=CARTESIAN_POINT('Ctrl Pts',(46.4891218839111,-18.2033415583671,72.8920641183648));
#3487=CARTESIAN_POINT('Ctrl Pts',(47.7818243197045,-20.9528181004838,73.2830212815669));
#3488=CARTESIAN_POINT('Ctrl Pts',(50.2187210719051,-22.7672877187656,73.6739784447688));
#3489=CARTESIAN_POINT('Ctrl Pts',(53.2234261185118,-23.2174195646428,74.0649356079709));
#3490=CARTESIAN_POINT('Ctrl Pts',(56.085013860659,-22.196986288013,74.4558927711729));
#3491=CARTESIAN_POINT('Ctrl Pts',(58.1268398486099,-19.9468301996286,74.846849934375));
#3492=CARTESIAN_POINT('Ctrl Pts',(58.6189035487885,-17.9825825214271,75.1074880431764));
#3493=CARTESIAN_POINT('Ctrl Pts',(58.6189035487885,-17.,75.237807097577));
#3494=CARTESIAN_POINT('',(56.6189035487885,-17.,75.2378070975771));
#3495=CARTESIAN_POINT('Ctrl Pts',(58.6189035487885,-17.,75.237807097577));
#3496=CARTESIAN_POINT('Ctrl Pts',(58.6189035487885,-17.008960117349,75.3053647907907));
#3497=CARTESIAN_POINT('Ctrl Pts',(58.6117944887821,-17.0178948508948,75.3727310946367));
#3498=CARTESIAN_POINT('Ctrl Pts',(58.5835895459723,-17.0354327396429,75.5049636605181));
#3499=CARTESIAN_POINT('Ctrl Pts',(58.5625652615718,-17.0439860715606,75.5694542638574));
#3500=CARTESIAN_POINT('Ctrl Pts',(58.4828049675281,-17.0676897484131,75.7481757768082));
#3501=CARTESIAN_POINT('Ctrl Pts',(58.4079637983781,-17.0816898329777,75.8537339275911));
#3502=CARTESIAN_POINT('Ctrl Pts',(58.2206375760899,-17.1052702229138,76.0315258790922));
#3503=CARTESIAN_POINT('Ctrl Pts',(58.1096236898478,-17.1145665084967,76.1016182210869));
#3504=CARTESIAN_POINT('Ctrl Pts',(57.8656078740837,-17.1271089995502,76.1961863756905));
#3505=CARTESIAN_POINT('Ctrl Pts',(57.7347565193837,-17.1301779251459,76.2193255295076));
#3506=CARTESIAN_POINT('Ctrl Pts',(57.4713951509218,-17.1295550490469,76.2146291543638));
#3507=CARTESIAN_POINT('Ctrl Pts',(57.3412656322973,-17.1258605590003,76.1867733556523));
#3508=CARTESIAN_POINT('Ctrl Pts',(57.1006247689232,-17.1122064533128,76.0838238241662));
#3509=CARTESIAN_POINT('Ctrl Pts',(56.9919980123763,-17.1024344565023,76.0101447038231));
#3510=CARTESIAN_POINT('Ctrl Pts',(56.8111979530795,-17.0781956792231,75.8273886287054));
#3511=CARTESIAN_POINT('Ctrl Pts',(56.7400261926721,-17.064034548912,75.7206162211305));
#3512=CARTESIAN_POINT('Ctrl Pts',(56.6436413373651,-17.0330811637281,75.4872331951366));
#3513=CARTESIAN_POINT('Ctrl Pts',(56.6189035487885,-17.0166298921152,75.3631935301346));
#3514=CARTESIAN_POINT('Ctrl Pts',(56.6189035487885,-17.,75.2378070975771));
#3515=CARTESIAN_POINT('',(56.7160709287438,-17.0505280490765,74.7973480456327));
#3516=CARTESIAN_POINT('Ctrl Pts',(56.619807216532,-17.,75.2373164241775));
#3517=CARTESIAN_POINT('Ctrl Pts',(56.6197919231519,-17.0008600414084,75.22926047205));
#3518=CARTESIAN_POINT('Ctrl Pts',(56.6198658096928,-17.0017200514272,75.2212050523955));
#3519=CARTESIAN_POINT('Ctrl Pts',(56.6200289121166,-17.0025803567058,75.2131518394368));
#3520=CARTESIAN_POINT('Ctrl Pts',(56.6209590323085,-17.0074863985172,75.1672269794184));
#3521=CARTESIAN_POINT('Ctrl Pts',(56.6247833784199,-17.0123852229216,75.1215182732402));
#3522=CARTESIAN_POINT('Ctrl Pts',(56.6314848898377,-17.0173394870174,75.0763314642167));
#3523=CARTESIAN_POINT('Ctrl Pts',(56.6380508197605,-17.0221935190177,75.0320588512208));
#3524=CARTESIAN_POINT('Ctrl Pts',(56.6473788385076,-17.027100631373,74.9882860750618));
#3525=CARTESIAN_POINT('Ctrl Pts',(56.659501419885,-17.0321210350159,74.9453059975962));
#3526=CARTESIAN_POINT('Ctrl Pts',(56.6674796286738,-17.0354251026249,74.9170196103077));
#3527=CARTESIAN_POINT('Ctrl Pts',(56.6766692322283,-17.0387782700352,74.8890767068547));
#3528=CARTESIAN_POINT('Ctrl Pts',(56.6870908888333,-17.0421984494337,74.8615656693999));
#3529=CARTESIAN_POINT('Ctrl Pts',(56.6954202403711,-17.0449319761283,74.8395778884914));
#3530=CARTESIAN_POINT('Ctrl Pts',(56.7045106227115,-17.0477003616562,74.8179350323125));
#3531=CARTESIAN_POINT('Ctrl Pts',(56.7143627134912,-17.0505136943971,74.7966769441347));
#3532=CARTESIAN_POINT('',(57.0485964548729,-16.9999999999999,74.4163755309633));
#3533=CARTESIAN_POINT('Ctrl Pts',(56.7160709287427,-17.0505280490768,74.7973480456349));
#3534=CARTESIAN_POINT('Ctrl Pts',(56.734112437174,-17.0456614403176,74.7606546800529));
#3535=CARTESIAN_POINT('Ctrl Pts',(56.7545070450986,-17.0409383108094,74.7250431225245));
#3536=CARTESIAN_POINT('Ctrl Pts',(56.8485610192468,-17.0220366934414,74.5825282850899));
#3537=CARTESIAN_POINT('Ctrl Pts',(56.9409174602205,-17.0096845848757,74.4893955806398));
#3538=CARTESIAN_POINT('Ctrl Pts',(57.048596454873,-17.,74.4163755309633));
#3539=CARTESIAN_POINT('',(58.1892106427041,-17.,74.4163755309633));
#3540=CARTESIAN_POINT('Origin',(57.6189035487885,-17.,75.237807097577));
#3541=CARTESIAN_POINT('Origin',(57.6189035487885,-17.,75.237807097577));
#3542=CARTESIAN_POINT('Ctrl Pts',(58.6189035487885,-17.,50.237807097577));
#3543=CARTESIAN_POINT('Ctrl Pts',(58.6189035487885,-16.991039882651,50.1702494043634));
#3544=CARTESIAN_POINT('Ctrl Pts',(58.6117944887821,-16.9821051491052,50.1028831005174));
#3545=CARTESIAN_POINT('Ctrl Pts',(58.5835895459723,-16.9645672603571,49.9706505346359));
#3546=CARTESIAN_POINT('Ctrl Pts',(58.5625652615718,-16.9560139284394,49.9061599312966));
#3547=CARTESIAN_POINT('Ctrl Pts',(58.4828049675281,-16.9323102515869,49.7274384183459));
#3548=CARTESIAN_POINT('Ctrl Pts',(58.4079637983781,-16.9183101670223,49.6218802675629));
#3549=CARTESIAN_POINT('Ctrl Pts',(58.2206375760899,-16.8947297770862,49.4440883160619));
#3550=CARTESIAN_POINT('Ctrl Pts',(58.1096236898478,-16.8854334915033,49.3739959740672));
#3551=CARTESIAN_POINT('Ctrl Pts',(57.8656078740836,-16.8728910004498,49.2794278194636));
#3552=CARTESIAN_POINT('Ctrl Pts',(57.7347565193837,-16.8698220748541,49.2562886656465));
#3553=CARTESIAN_POINT('Ctrl Pts',(57.4713951509218,-16.8704449509531,49.2609850407903));
#3554=CARTESIAN_POINT('Ctrl Pts',(57.3412656322973,-16.8741394409997,49.2888408395018));
#3555=CARTESIAN_POINT('Ctrl Pts',(57.1006247689232,-16.8877935466872,49.3917903709879));
#3556=CARTESIAN_POINT('Ctrl Pts',(56.9919980123763,-16.8975655434977,49.465469491331));
#3557=CARTESIAN_POINT('Ctrl Pts',(56.8111979530794,-16.9218043207769,49.6482255664488));
#3558=CARTESIAN_POINT('Ctrl Pts',(56.740026192672,-16.935965451088,49.7549979740236));
#3559=CARTESIAN_POINT('Ctrl Pts',(56.6436413373651,-16.9669188362719,49.9883810000176));
#3560=CARTESIAN_POINT('Ctrl Pts',(56.6189035487885,-16.9833701078848,50.1124206650196));
#3561=CARTESIAN_POINT('Ctrl Pts',(56.6189035487885,-17.,50.237807097577));
#3562=CARTESIAN_POINT('Origin',(57.6189035487885,-17.15,50.237807097577));
#3563=CARTESIAN_POINT('Ctrl Pts',(57.0353881436569,-17.1499999999404,49.3968642735725));
#3564=CARTESIAN_POINT('Ctrl Pts',(56.9995277725034,-17.1500003183691,49.4222269403983));
#3565=CARTESIAN_POINT('Ctrl Pts',(56.9653733978866,-17.1500025402159,49.4500582165395));
#3566=CARTESIAN_POINT('Ctrl Pts',(56.9331114218803,-17.1500046663948,49.4801422563167));
#3567=CARTESIAN_POINT('Ctrl Pts',(56.9007444405485,-17.1500067994939,49.5103242127372));
#3568=CARTESIAN_POINT('Ctrl Pts',(56.8704989342592,-17.1500088846928,49.5425711070994));
#3569=CARTESIAN_POINT('Ctrl Pts',(56.842517628275,-17.1500096437477,49.576616148902));
#3570=CARTESIAN_POINT('Ctrl Pts',(56.8144621758977,-17.1500104048139,49.6107514051163));
#3571=CARTESIAN_POINT('Ctrl Pts',(56.7886822426408,-17.1500098407062,49.646695273018));
#3572=CARTESIAN_POINT('Ctrl Pts',(56.7653583390214,-17.1500083475778,49.6842152192191));
#3573=CARTESIAN_POINT('Ctrl Pts',(56.7440381590042,-17.1500069827219,49.7185118798595));
#3574=CARTESIAN_POINT('Ctrl Pts',(56.7247701610183,-17.1500048688239,49.7541263894184));
#3575=CARTESIAN_POINT('Ctrl Pts',(56.7077264766587,-17.1500034254948,49.7908978528519));
#3576=CARTESIAN_POINT('Ctrl Pts',(56.6967102134416,-17.1500024925924,49.8146652561618));
#3577=CARTESIAN_POINT('Ctrl Pts',(56.6866679969386,-17.1500013277767,49.8388214631241));
#3578=CARTESIAN_POINT('Ctrl Pts',(56.6776310476167,-17.1500011365132,49.863315773977));
#3579=CARTESIAN_POINT('Ctrl Pts',(56.6624572664577,-17.150000815366,49.9044437364435));
#3580=CARTESIAN_POINT('Ctrl Pts',(56.650114799487,-17.1500032648176,49.9465239883955));
#3581=CARTESIAN_POINT('Ctrl Pts',(56.640580505364,-17.1500062417895,49.9892605406622));
#3582=CARTESIAN_POINT('Ctrl Pts',(56.6309401368815,-17.150009251882,50.0324725609973));
#3583=CARTESIAN_POINT('Ctrl Pts',(56.624170610253,-17.1500128171849,50.0763567021812));
#3584=CARTESIAN_POINT('Ctrl Pts',(56.6202990237812,-17.1500140834455,50.1206190671135));
#3585=CARTESIAN_POINT('Ctrl Pts',(56.6190338326219,-17.1500144972454,50.1350835129449));
#3586=CARTESIAN_POINT('Ctrl Pts',(56.6180785278747,-17.1500146602173,50.1495883714516));
#3587=CARTESIAN_POINT('Ctrl Pts',(56.6174352663666,-17.1500144553777,50.1641233425841));
#3588=CARTESIAN_POINT('Ctrl Pts',(56.6154669730407,-17.150013828596,50.2085983909243));
#3589=CARTESIAN_POINT('Ctrl Pts',(56.6164293147499,-17.1500098830758,50.2530643615513));
#3590=CARTESIAN_POINT('Ctrl Pts',(56.6203035167127,-17.1500063372223,50.2972233337701));
#3591=CARTESIAN_POINT('Ctrl Pts',(56.6241712235008,-17.1500027973134,50.3413082726175));
#3592=CARTESIAN_POINT('Ctrl Pts',(56.6309410033718,-17.1499996436082,50.3850883978143));
#3593=CARTESIAN_POINT('Ctrl Pts',(56.6406452513128,-17.1499996640019,50.4282695972847));
#3594=CARTESIAN_POINT('Ctrl Pts',(56.6424167756711,-17.1499996677248,50.4361523870845));
#3595=CARTESIAN_POINT('Ctrl Pts',(56.6442862295108,-17.1499997750282,50.4440151968179));
#3596=CARTESIAN_POINT('Ctrl Pts',(56.6462539958365,-17.1499999999996,50.4518561987028));
#3597=CARTESIAN_POINT('Origin',(57.6189035487885,-17.,75.237807097577));
#3598=CARTESIAN_POINT('',(58.1993466393407,-17.,74.4163755309629));
#3599=CARTESIAN_POINT('',(57.6189035487885,-17.,74.4163755309633));
#3600=CARTESIAN_POINT('Ctrl Pts',(58.1997282611953,-16.9998571535648,74.4152984942148));
#3601=CARTESIAN_POINT('Ctrl Pts',(58.2143357917363,-16.9998440707738,74.4257197573308));
#3602=CARTESIAN_POINT('Ctrl Pts',(58.2286519425552,-16.9998332935578,74.4365601307609));
#3603=CARTESIAN_POINT('Ctrl Pts',(58.2426546458167,-16.9998261318276,74.4478189175199));
#3604=CARTESIAN_POINT('Ctrl Pts',(58.2570875587164,-16.9998187500652,74.4594236116718));
#3605=CARTESIAN_POINT('Ctrl Pts',(58.271187472638,-16.9998152116138,74.4714728412125));
#3606=CARTESIAN_POINT('Ctrl Pts',(58.2849450357921,-16.9998144462796,74.4839469418765));
#3607=CARTESIAN_POINT('Ctrl Pts',(58.3171667594867,-16.999812653783,74.5131626554759));
#3608=CARTESIAN_POINT('Ctrl Pts',(58.3473079189655,-16.9998260898473,74.544520126789));
#3609=CARTESIAN_POINT('Ctrl Pts',(58.3753004444692,-16.9998438498395,74.5777107138075));
#3610=CARTESIAN_POINT('Ctrl Pts',(58.4041614873196,-16.9998621608667,74.6119310971753));
#3611=CARTESIAN_POINT('Ctrl Pts',(58.4307391732154,-16.9998851867719,74.6481009779077));
#3612=CARTESIAN_POINT('Ctrl Pts',(58.4549224048529,-16.9999065586214,74.685924045946));
#3613=CARTESIAN_POINT('Ctrl Pts',(58.4775163765478,-16.9999265259678,74.7212614789856));
#3614=CARTESIAN_POINT('Ctrl Pts',(58.4980202826146,-16.9999452002503,74.7580430626991));
#3615=CARTESIAN_POINT('Ctrl Pts',(58.5163082288499,-16.9999601156304,74.7960480062526));
#3616=CARTESIAN_POINT('Ctrl Pts',(58.5359309705969,-16.9999761196501,74.8368268440109));
#3617=CARTESIAN_POINT('Ctrl Pts',(58.5528792611933,-16.9999879520546,74.8787568015286));
#3618=CARTESIAN_POINT('Ctrl Pts',(58.5670508442818,-16.9999950681616,74.9215394899968));
#3619=CARTESIAN_POINT('Ctrl Pts',(58.5810408703955,-17.0000020931016,74.9637740748802));
#3620=CARTESIAN_POINT('Ctrl Pts',(58.5923252734734,-17.000004670778,75.0068407878673));
#3621=CARTESIAN_POINT('Ctrl Pts',(58.600760876798,-17.0000048908046,75.0504735477835));
#3622=CARTESIAN_POINT('Ctrl Pts',(58.6087537841981,-17.0000050992843,75.0918164839313));
#3623=CARTESIAN_POINT('Ctrl Pts',(58.6141890828729,-17.0000033086596,75.1336685099678));
#3624=CARTESIAN_POINT('Ctrl Pts',(58.6169020048606,-17.0000017472687,75.175807863164));
#3625=CARTESIAN_POINT('Ctrl Pts',(58.6182322861701,-17.0000009816407,75.1964708952038));
#3626=CARTESIAN_POINT('Ctrl Pts',(58.6189035487885,-16.999997221476,75.2171455663987));
#3627=CARTESIAN_POINT('Ctrl Pts',(58.6189035487885,-17.0000000161406,75.2378038846518));
#3628=CARTESIAN_POINT('Ctrl Pts',(58.6189035487885,-17.1070624647046,75.2236074971792));
#3629=CARTESIAN_POINT('Ctrl Pts',(58.6189035487885,-17.0713749764698,75.2283406973118));
#3630=CARTESIAN_POINT('Ctrl Pts',(58.6189035487885,-17.0356873793413,75.2330738853036));
#3631=CARTESIAN_POINT('Ctrl Pts',(58.6189035487885,-16.868940610655,75.2551744844083));
#3632=CARTESIAN_POINT('Ctrl Pts',(58.6189035487886,-16.6072943602623,75.2878910531892));
#3633=CARTESIAN_POINT('Ctrl Pts',(58.6189035487885,-16.0863108570333,75.3474872987329));
#3634=CARTESIAN_POINT('Ctrl Pts',(58.6189035487885,-15.4407089605501,75.4198407374667));
#3635=CARTESIAN_POINT('Ctrl Pts',(58.6189035487886,-14.810515552782,75.530562741844));
#3636=CARTESIAN_POINT('Ctrl Pts',(58.6189035487885,-14.3226785985763,75.6740330751718));
#3637=CARTESIAN_POINT('Ctrl Pts',(58.6189035487886,-13.6119901077366,75.9531021796814));
#3638=CARTESIAN_POINT('Ctrl Pts',(58.6189035487885,-12.6391386971879,76.6898853504872));
#3639=CARTESIAN_POINT('Ctrl Pts',(58.6189035487886,-11.9421053181931,77.9551448661809));
#3640=CARTESIAN_POINT('Ctrl Pts',(58.6189035487886,-11.620123611833,78.904610366011));
#3641=CARTESIAN_POINT('Ctrl Pts',(58.6189035487886,-11.4414090651326,79.5566822517067));
#3642=CARTESIAN_POINT('Ctrl Pts',(58.6189035487886,-11.283611680672,80.3904836204666));
#3643=CARTESIAN_POINT('Ctrl Pts',(58.6189035487885,-11.191771906312,81.2094324300899));
#3644=CARTESIAN_POINT('Ctrl Pts',(58.6189035487885,-11.1351578812696,81.8374901150816));
#3645=CARTESIAN_POINT('Ctrl Pts',(58.6189035487885,-11.053369822089,82.7460850644104));
#3646=CARTESIAN_POINT('Ctrl Pts',(58.6189035487885,-10.9236831233095,83.6860531538696));
#3647=CARTESIAN_POINT('Ctrl Pts',(58.6189035487885,-10.4992473440377,84.5353425071605));
#3648=CARTESIAN_POINT('Ctrl Pts',(58.6189035487886,-10.0852341421502,84.9682405076987));
#3649=CARTESIAN_POINT('Ctrl Pts',(58.6189035487886,-9.65205447547462,85.2538515396933));
#3650=CARTESIAN_POINT('Ctrl Pts',(58.6189035487886,-9.1488264052405,85.4990822689984));
#3651=CARTESIAN_POINT('Ctrl Pts',(58.6189035487885,-8.07907491053992,85.8217946659718));
#3652=CARTESIAN_POINT('Ctrl Pts',(58.6189035487885,-6.83128625461351,85.9175112317093));
#3653=CARTESIAN_POINT('Ctrl Pts',(58.6189035487885,-5.85324890998301,85.9023446784181));
#3654=CARTESIAN_POINT('Ctrl Pts',(58.6189035487885,-17.0677244044812,74.9270055107683));
#3655=CARTESIAN_POINT('Ctrl Pts',(58.6189035487885,-17.0320369162463,74.9317387109009));
#3656=CARTESIAN_POINT('Ctrl Pts',(58.6189035487885,-16.9963437059072,74.9364726710977));
#3657=CARTESIAN_POINT('Ctrl Pts',(58.6189035487885,-16.8296431542228,74.9585653195626));
#3658=CARTESIAN_POINT('Ctrl Pts',(58.6189035487886,-16.5713180684596,74.990859086523));
#3659=CARTESIAN_POINT('Ctrl Pts',(58.6189035487885,-16.0526651090702,75.050198376707));
#3660=CARTESIAN_POINT('Ctrl Pts',(58.6189035487885,-15.40137640994,75.1231150129893));
#3661=CARTESIAN_POINT('Ctrl Pts',(58.6189035487886,-14.7450284330187,75.2377433098845));
#3662=CARTESIAN_POINT('Ctrl Pts',(58.6189035487885,-14.2255085991446,75.3905130433138));
#3663=CARTESIAN_POINT('Ctrl Pts',(58.6189035487886,-13.4573378756898,75.691187535415));
#3664=CARTESIAN_POINT('Ctrl Pts',(58.6189035487885,-12.3965385704437,76.4991688124884));
#3665=CARTESIAN_POINT('Ctrl Pts',(58.6189035487886,-11.6684548706516,77.8319408520014));
#3666=CARTESIAN_POINT('Ctrl Pts',(58.6189035487886,-11.3339319292239,78.8171580204204));
#3667=CARTESIAN_POINT('Ctrl Pts',(58.6189035487886,-11.1493868708181,79.4910278264843));
#3668=CARTESIAN_POINT('Ctrl Pts',(58.6189035487886,-10.9873493355326,80.347370825992));
#3669=CARTESIAN_POINT('Ctrl Pts',(58.6189035487885,-10.8941820327677,81.1800702256411));
#3670=CARTESIAN_POINT('Ctrl Pts',(58.6189035487885,-10.8371602227307,81.8111085619185));
#3671=CARTESIAN_POINT('Ctrl Pts',(58.6189035487885,-10.7562651177072,82.7152910391538));
#3672=CARTESIAN_POINT('Ctrl Pts',(58.6189035487885,-10.62680068035,83.6154368879388));
#3673=CARTESIAN_POINT('Ctrl Pts',(58.6189035487885,-10.2493987285943,84.3618958202144));
#3674=CARTESIAN_POINT('Ctrl Pts',(58.6189035487886,-9.8919152225634,84.7369092153924));
#3675=CARTESIAN_POINT('Ctrl Pts',(58.6189035487886,-9.50503348466235,84.9925351153733));
#3676=CARTESIAN_POINT('Ctrl Pts',(58.6189035487886,-9.04537663272557,85.2168574142422));
#3677=CARTESIAN_POINT('Ctrl Pts',(58.6189035487885,-8.0378464978853,85.5227638874191));
#3678=CARTESIAN_POINT('Ctrl Pts',(58.6189035487885,-6.82025743271601,85.6181049337487));
#3679=CARTESIAN_POINT('Ctrl Pts',(58.6189035487885,-5.85788807498938,85.603181345984));
#3680=CARTESIAN_POINT('Ctrl Pts',(58.3322714066286,-16.9892828575829,74.3355701808357));
#3681=CARTESIAN_POINT('Ctrl Pts',(58.3322714066286,-16.953595369348,74.3403033809683));
#3682=CARTESIAN_POINT('Ctrl Pts',(58.3322714066287,-16.9178909302647,74.3450389025498));
#3683=CARTESIAN_POINT('Ctrl Pts',(58.3322714066286,-16.7512842541308,74.3671145332137));
#3684=CARTESIAN_POINT('Ctrl Pts',(58.3322714066287,-16.499588634895,74.3985624655087));
#3685=CARTESIAN_POINT('Ctrl Pts',(58.3322714066286,-15.9855939784622,74.4573831305653));
#3686=CARTESIAN_POINT('Ctrl Pts',(58.3322714066287,-15.3229750899196,74.5314130013934));
#3687=CARTESIAN_POINT('Ctrl Pts',(58.3322714066287,-14.6144661000659,74.6538202774898));
#3688=CARTESIAN_POINT('Ctrl Pts',(58.3322714066287,-14.0317403735836,74.8251403710485));
#3689=CARTESIAN_POINT('Ctrl Pts',(58.3322714066287,-13.148909444107,75.1689004861853));
#3690=CARTESIAN_POINT('Ctrl Pts',(58.3322714066286,-11.9126649225552,76.1189177484811));
#3691=CARTESIAN_POINT('Ctrl Pts',(58.3322714066287,-11.1227142479736,77.5862953260158));
#3692=CARTESIAN_POINT('Ctrl Pts',(58.3322714066287,-10.7631722715652,78.642838701811));
#3693=CARTESIAN_POINT('Ctrl Pts',(58.3322714066287,-10.5669977147391,79.3601938732302));
#3694=CARTESIAN_POINT('Ctrl Pts',(58.3322714066287,-10.3965037381347,80.2615040278716));
#3695=CARTESIAN_POINT('Ctrl Pts',(58.3322714066286,-10.3006886617217,81.1216343338287));
#3696=CARTESIAN_POINT('Ctrl Pts',(58.3322714066286,-10.2428505130289,81.7586216789515));
#3697=CARTESIAN_POINT('Ctrl Pts',(58.3322714066286,-10.1637401686721,82.6539973819218));
#3698=CARTESIAN_POINT('Ctrl Pts',(58.3322714066287,-10.0346447578536,83.4747687679503));
#3699=CARTESIAN_POINT('Ctrl Pts',(58.3322714066287,-9.75107986379657,84.0160716707905));
#3700=CARTESIAN_POINT('Ctrl Pts',(58.3322714066287,-9.50634793399624,84.2756235640084));
#3701=CARTESIAN_POINT('Ctrl Pts',(58.3322714066287,-9.2118265761089,84.4714332158408));
#3702=CARTESIAN_POINT('Ctrl Pts',(58.3322714066287,-8.83908636867753,84.6540485794195));
#3703=CARTESIAN_POINT('Ctrl Pts',(58.3322714066287,-7.9556774348701,84.9264368884188));
#3704=CARTESIAN_POINT('Ctrl Pts',(58.3322714066286,-6.79824855322479,85.0210774392432));
#3705=CARTESIAN_POINT('Ctrl Pts',(58.3322714066286,-5.86713874157915,85.0066385973567));
#3706=CARTESIAN_POINT('Ctrl Pts',(57.3646226285175,-16.9604946724078,74.1185123783007));
#3707=CARTESIAN_POINT('Ctrl Pts',(57.3646226285175,-16.9248071841729,74.1232455784333));
#3708=CARTESIAN_POINT('Ctrl Pts',(57.3646226285175,-16.889098333514,74.1279818482412));
#3709=CARTESIAN_POINT('Ctrl Pts',(57.3646226285175,-16.7225400508609,74.1500417837015));
#3710=CARTESIAN_POINT('Ctrl Pts',(57.3646226285175,-16.4733338130514,74.1811569488366));
#3711=CARTESIAN_POINT('Ctrl Pts',(57.3646226285175,-15.9611389801221,74.2397365628143));
#3712=CARTESIAN_POINT('Ctrl Pts',(57.3646226285175,-15.2944390637735,74.3140954113275));
#3713=CARTESIAN_POINT('Ctrl Pts',(57.3646226285175,-14.5667232822858,74.4392738616914));
#3714=CARTESIAN_POINT('Ctrl Pts',(57.3646226285175,-13.9605649616208,74.6174589018033));
#3715=CARTESIAN_POINT('Ctrl Pts',(57.3646226285176,-13.0353408967044,74.9770614024389));
#3716=CARTESIAN_POINT('Ctrl Pts',(57.3646226285175,-11.7341080097852,75.9797283837915));
#3717=CARTESIAN_POINT('Ctrl Pts',(57.3646226285176,-10.9218459124412,77.4963689695129));
#3718=CARTESIAN_POINT('Ctrl Pts',(57.3646226285176,-10.5530297713597,78.5793819337369));
#3719=CARTESIAN_POINT('Ctrl Pts',(57.3646226285175,-10.3525608436317,79.312854674376));
#3720=CARTESIAN_POINT('Ctrl Pts',(57.3646226285176,-10.1789517790958,80.2308165058766));
#3721=CARTESIAN_POINT('Ctrl Pts',(57.3646226285175,-10.0821598266619,81.1011091643012));
#3722=CARTESIAN_POINT('Ctrl Pts',(57.3646226285175,-10.023996097922,81.7403242963189));
#3723=CARTESIAN_POINT('Ctrl Pts',(57.3646226285175,-9.94557467621999,82.6324017972352));
#3724=CARTESIAN_POINT('Ctrl Pts',(57.3646226285175,-9.81601252498804,83.4243069447849));
#3725=CARTESIAN_POINT('Ctrl Pts',(57.3646226285175,-9.56729084574229,83.8894374229533));
#3726=CARTESIAN_POINT('Ctrl Pts',(57.3646226285175,-9.36417659416019,84.1063106299724));
#3727=CARTESIAN_POINT('Ctrl Pts',(57.3646226285175,-9.10388126033771,84.2799663831815));
#3728=CARTESIAN_POINT('Ctrl Pts',(57.3646226285175,-8.76331584417413,84.4471554629121));
#3729=CARTESIAN_POINT('Ctrl Pts',(57.3646226285175,-7.92586155372296,84.7071895267139));
#3730=CARTESIAN_POINT('Ctrl Pts',(57.3646226285175,-6.79003323137325,84.8019651621459));
#3731=CARTESIAN_POINT('Ctrl Pts',(57.3646226285175,-5.87053375242876,84.7877063632102));
#3732=CARTESIAN_POINT('Ctrl Pts',(56.5859422264137,-17.0417044640364,74.7308197817729));
#3733=CARTESIAN_POINT('Ctrl Pts',(56.5859422264137,-17.0060169758015,74.7355529819055));
#3734=CARTESIAN_POINT('Ctrl Pts',(56.5859422264137,-16.9703200156519,74.7402874751691));
#3735=CARTESIAN_POINT('Ctrl Pts',(56.5859422264137,-16.8036518081296,74.7623736621299));
#3736=CARTESIAN_POINT('Ctrl Pts',(56.5859422264137,-16.5475306602109,74.7943849255561));
#3737=CARTESIAN_POINT('Ctrl Pts',(56.5859422264137,-16.0304307075519,74.8535477998962));
#3738=CARTESIAN_POINT('Ctrl Pts',(56.5859422264137,-15.3753903256926,74.926826832225));
#3739=CARTESIAN_POINT('Ctrl Pts',(56.5859422264137,-14.7017344598755,75.0440282693776));
#3740=CARTESIAN_POINT('Ctrl Pts',(56.5859422264137,-14.1612281378247,75.2029562844881));
#3741=CARTESIAN_POINT('Ctrl Pts',(56.5859422264137,-13.3549963246989,75.517925343114));
#3742=CARTESIAN_POINT('Ctrl Pts',(56.5859422264136,-12.2359480597188,76.3730666756037));
#3743=CARTESIAN_POINT('Ctrl Pts',(56.5859422264138,-11.4873764233173,77.7504770035942));
#3744=CARTESIAN_POINT('Ctrl Pts',(56.5859422264137,-11.1445464264738,78.7593791696242));
#3745=CARTESIAN_POINT('Ctrl Pts',(56.5859422264137,-10.9561414584619,79.4476872424981));
#3746=CARTESIAN_POINT('Ctrl Pts',(56.5859422264137,-10.7912978280097,80.3189591959352));
#3747=CARTESIAN_POINT('Ctrl Pts',(56.5859422264137,-10.6972517850491,81.1607659572902));
#3748=CARTESIAN_POINT('Ctrl Pts',(56.5859422264137,-10.6399569412909,81.7937814907276));
#3749=CARTESIAN_POINT('Ctrl Pts',(56.5859422264137,-10.5596567916307,82.6950369507156));
#3750=CARTESIAN_POINT('Ctrl Pts',(56.5859422264137,-10.4302627328852,83.5688762400591));
#3751=CARTESIAN_POINT('Ctrl Pts',(56.5859422264137,-10.0840225667115,84.2472065970568));
#3752=CARTESIAN_POINT('Ctrl Pts',(56.5859422264137,-9.76396055712458,84.5838938404408));
#3753=CARTESIAN_POINT('Ctrl Pts',(56.5859422264137,-9.40774427240785,84.8196606327552));
#3754=CARTESIAN_POINT('Ctrl Pts',(56.5859422264137,-8.97694251385567,85.0301379251509));
#3755=CARTESIAN_POINT('Ctrl Pts',(56.5859422264137,-8.01061950340817,85.3249214662463));
#3756=CARTESIAN_POINT('Ctrl Pts',(56.5859422264137,-6.81294491447546,85.4200640361347));
#3757=CARTESIAN_POINT('Ctrl Pts',(56.5859422264137,-5.86095662479822,85.4053014289528));
#3758=CARTESIAN_POINT('Ctrl Pts',(56.5889518727976,-17.1722671939372,75.7152395731868));
#3759=CARTESIAN_POINT('Ctrl Pts',(56.5889518727976,-17.1365797057023,75.7199727733194));
#3760=CARTESIAN_POINT('Ctrl Pts',(56.5889518727976,-17.1009015634799,75.7247045904694));
#3761=CARTESIAN_POINT('Ctrl Pts',(56.5889518727976,-16.9340709566345,75.7468232697129));
#3762=CARTESIAN_POINT('Ctrl Pts',(56.5889518727976,-16.6668904840349,75.7802522429883));
#3763=CARTESIAN_POINT('Ctrl Pts',(56.5889518727976,-16.1419971956025,75.8403007103795));
#3764=CARTESIAN_POINT('Ctrl Pts',(56.5889518727976,-15.5057814191354,75.9117619012503));
#3765=CARTESIAN_POINT('Ctrl Pts',(56.5889518727976,-14.9189734632704,76.0160524660517));
#3766=CARTESIAN_POINT('Ctrl Pts',(56.5889518727976,-14.4837747810549,76.144079065061));
#3767=CARTESIAN_POINT('Ctrl Pts',(56.5889518727976,-13.8685280261394,76.387320697005));
#3768=CARTESIAN_POINT('Ctrl Pts',(56.5889518727976,-13.0417655345062,77.0058186775411));
#3769=CARTESIAN_POINT('Ctrl Pts',(56.5889518727977,-12.395995257802,78.1592442349785));
#3770=CARTESIAN_POINT('Ctrl Pts',(56.5889518727976,-12.0948490433455,79.0492977741235));
#3771=CARTESIAN_POINT('Ctrl Pts',(56.5889518727976,-11.9258125052654,79.6651564130096));
#3772=CARTESIAN_POINT('Ctrl Pts',(56.5889518727976,-11.7750493707723,80.4615168367482));
#3773=CARTESIAN_POINT('Ctrl Pts',(56.5889518727976,-11.6854127040116,81.2576240203752));
#3774=CARTESIAN_POINT('Ctrl Pts',(56.5889518727976,-11.629488079385,81.8807180550451));
#3775=CARTESIAN_POINT('Ctrl Pts',(56.5889518727976,-11.5462023151942,82.7966611759654));
#3776=CARTESIAN_POINT('Ctrl Pts',(56.5889518727976,-11.4164595576202,83.802499438733));
#3777=CARTESIAN_POINT('Ctrl Pts',(56.5889518727976,-10.9138529466339,84.8226915242591));
#3778=CARTESIAN_POINT('Ctrl Pts',(56.5889518727976,-10.4060157803267,85.3516937903176));
#3779=CARTESIAN_POINT('Ctrl Pts',(56.5889518727976,-9.89592410072379,85.6871110018963));
#3780=CARTESIAN_POINT('Ctrl Pts',(56.5889518727976,-9.32033135595104,85.9670605844408));
#3781=CARTESIAN_POINT('Ctrl Pts',(56.5889518727976,-8.14723647018877,86.3176571112496));
#3782=CARTESIAN_POINT('Ctrl Pts',(56.5889518727976,-6.84963865195032,86.4137926993747));
#3783=CARTESIAN_POINT('Ctrl Pts',(56.5889518727976,-5.8455592705756,86.3982223088065));
#3784=CARTESIAN_POINT('Ctrl Pts',(57.3635556629615,-17.2540588078706,76.331933813487));
#3785=CARTESIAN_POINT('Ctrl Pts',(57.3635556629615,-17.2183713196357,76.3366670136196));
#3786=CARTESIAN_POINT('Ctrl Pts',(57.3635556629615,-17.1827047092038,76.3413973091119));
#3787=CARTESIAN_POINT('Ctrl Pts',(57.3635556629615,-17.0157846850654,76.3635279934273));
#3788=CARTESIAN_POINT('Ctrl Pts',(57.3635556629616,-16.7417258451673,76.3978253536053));
#3789=CARTESIAN_POINT('Ctrl Pts',(57.3635556629615,-16.2120301045359,76.4583837923497));
#3790=CARTESIAN_POINT('Ctrl Pts',(57.3635556629615,-15.5876752775676,76.5286358687495));
#3791=CARTESIAN_POINT('Ctrl Pts',(57.3635556629616,-15.0552173829869,76.6247643784278));
#3792=CARTESIAN_POINT('Ctrl Pts',(57.3635556629615,-14.6857806853406,76.7334829512476));
#3793=CARTESIAN_POINT('Ctrl Pts',(57.3635556629616,-14.1899011326692,76.931817019722));
#3794=CARTESIAN_POINT('Ctrl Pts',(57.3635556629615,-13.5457125155092,77.4025301809331));
#3795=CARTESIAN_POINT('Ctrl Pts',(57.3635556629616,-12.9646906428169,78.4155180014605));
#3796=CARTESIAN_POINT('Ctrl Pts',(57.3635556629616,-12.6895760107024,79.2313769544293));
#3797=CARTESIAN_POINT('Ctrl Pts',(57.3635556629616,-12.5326496524696,79.8019892501139));
#3798=CARTESIAN_POINT('Ctrl Pts',(57.3635556629616,-12.3906970946281,80.5515523581134));
#3799=CARTESIAN_POINT('Ctrl Pts',(57.3635556629615,-12.3038181611488,81.3191149207297));
#3800=CARTESIAN_POINT('Ctrl Pts',(57.3635556629615,-12.2487289580723,81.9360328998565));
#3801=CARTESIAN_POINT('Ctrl Pts',(57.3635556629615,-12.1636028076754,82.8611187650277));
#3802=CARTESIAN_POINT('Ctrl Pts',(57.3635556629616,-12.033109514969,83.9498819481789));
#3803=CARTESIAN_POINT('Ctrl Pts',(57.3635556629615,-11.4329041685087,85.1834574545092));
#3804=CARTESIAN_POINT('Ctrl Pts',(57.3635556629616,-10.8076443977132,85.8326676190244));
#3805=CARTESIAN_POINT('Ctrl Pts',(57.3635556629616,-10.2014480222085,86.2303334764776));
#3806=CARTESIAN_POINT('Ctrl Pts',(57.3635556629616,-9.53539438980938,86.5536984632034));
#3807=CARTESIAN_POINT('Ctrl Pts',(57.3635556629615,-8.23312149114545,86.9392124383196));
#3808=CARTESIAN_POINT('Ctrl Pts',(57.3635556629615,-6.87250364926861,87.0363166333609));
#3809=CARTESIAN_POINT('Ctrl Pts',(57.3635556629615,-5.83591352823298,87.0202420944917));
#3810=CARTESIAN_POINT('Ctrl Pts',(58.3323903227877,-17.2245457788052,76.109410816774));
#3811=CARTESIAN_POINT('Ctrl Pts',(58.3323903227877,-17.1888582905703,76.1141440169066));
#3812=CARTESIAN_POINT('Ctrl Pts',(58.3323903227877,-17.1531877443463,76.1188747256693));
#3813=CARTESIAN_POINT('Ctrl Pts',(58.3323903227877,-16.9862891793002,76.1410084024959));
#3814=CARTESIAN_POINT('Ctrl Pts',(58.3323903227877,-16.714668593541,76.1750097398116));
#3815=CARTESIAN_POINT('Ctrl Pts',(58.3323903227877,-16.1866358039734,76.2354234730982));
#3816=CARTESIAN_POINT('Ctrl Pts',(58.3323903227877,-15.5579413523181,76.3061735193807));
#3817=CARTESIAN_POINT('Ctrl Pts',(58.3323903227877,-15.0059215204494,76.4053120537038));
#3818=CARTESIAN_POINT('Ctrl Pts',(58.3323903227877,-14.6129386564044,76.5209534522761));
#3819=CARTESIAN_POINT('Ctrl Pts',(58.3323903227877,-14.0742299245444,76.735468440667));
#3820=CARTESIAN_POINT('Ctrl Pts',(58.3323903227877,-13.3646276102391,77.2591022877258));
#3821=CARTESIAN_POINT('Ctrl Pts',(58.3323903227878,-12.7599371622137,78.3228710773516));
#3822=CARTESIAN_POINT('Ctrl Pts',(58.3323903227877,-12.4755009159366,79.165274904841));
#3823=CARTESIAN_POINT('Ctrl Pts',(58.3323903227877,-12.3142252216136,79.7520907812665));
#3824=CARTESIAN_POINT('Ctrl Pts',(58.3323903227877,-12.1691024854386,80.5184246380073));
#3825=CARTESIAN_POINT('Ctrl Pts',(58.3323903227877,-12.0812324563949,81.29621325344));
#3826=CARTESIAN_POINT('Ctrl Pts',(58.3323903227877,-12.0258619451679,81.9153252669056));
#3827=CARTESIAN_POINT('Ctrl Pts',(58.3323903227877,-11.9413735798053,82.8371633715007));
#3828=CARTESIAN_POINT('Ctrl Pts',(58.3323903227877,-11.8116178432401,83.8957997139702));
#3829=CARTESIAN_POINT('Ctrl Pts',(58.3323903227877,-11.2463154451697,85.0530615867849));
#3830=CARTESIAN_POINT('Ctrl Pts',(58.3323903227877,-10.6632413020241,85.6591326134248));
#3831=CARTESIAN_POINT('Ctrl Pts',(58.3323903227877,-10.0914671012367,86.0344931414346));
#3832=CARTESIAN_POINT('Ctrl Pts',(58.3323903227877,-9.45784054547688,86.3422852914887));
#3833=CARTESIAN_POINT('Ctrl Pts',(58.3323903227877,-8.20186765977983,86.7152410304432));
#3834=CARTESIAN_POINT('Ctrl Pts',(58.3323903227877,-6.86436020873407,86.8116917557747));
#3835=CARTESIAN_POINT('Ctrl Pts',(58.3323903227877,-5.83939402043047,86.7957974707539));
#3836=CARTESIAN_POINT('Ctrl Pts',(58.6189035487885,-17.1464005249281,75.5202094835902));
#3837=CARTESIAN_POINT('Ctrl Pts',(58.6189035487885,-17.1107130366932,75.5249426837228));
#3838=CARTESIAN_POINT('Ctrl Pts',(58.6189035487885,-17.0750310537087,75.5296750989469));
#3839=CARTESIAN_POINT('Ctrl Pts',(58.6189035487885,-16.9082380232507,75.5517836790378));
#3840=CARTESIAN_POINT('Ctrl Pts',(58.6189035487886,-16.6432704272489,75.5849231213956));
#3841=CARTESIAN_POINT('Ctrl Pts',(58.6189035487885,-16.119956090455,75.6447764851635));
#3842=CARTESIAN_POINT('Ctrl Pts',(58.6189035487885,-15.480040748791,75.7165669819153));
#3843=CARTESIAN_POINT('Ctrl Pts',(58.6189035487886,-14.8760021144475,75.8233829626469));
#3844=CARTESIAN_POINT('Ctrl Pts',(58.6189035487885,-14.419848797543,75.9575537130432));
#3845=CARTESIAN_POINT('Ctrl Pts',(58.6189035487886,-13.7666435433224,76.2150173339846));
#3846=CARTESIAN_POINT('Ctrl Pts',(58.6189035487885,-12.8817419532219,76.8806007213331));
#3847=CARTESIAN_POINT('Ctrl Pts',(58.6189035487886,-12.2157576301709,78.0783481546451));
#3848=CARTESIAN_POINT('Ctrl Pts',(58.6189035487886,-11.9063174547593,78.9920610457681));
#3849=CARTESIAN_POINT('Ctrl Pts',(58.6189035487886,-11.7334335043027,79.6223345025279));
#3850=CARTESIAN_POINT('Ctrl Pts',(58.6189035487886,-11.5798763077878,80.4335937631608));
#3851=CARTESIAN_POINT('Ctrl Pts',(58.6189035487885,-11.4893640783344,81.238791677157));
#3852=CARTESIAN_POINT('Ctrl Pts',(58.6189035487885,-11.4331579217258,81.8638685679878));
#3853=CARTESIAN_POINT('Ctrl Pts',(58.6189035487885,-11.3504767994824,82.776876201684));
#3854=CARTESIAN_POINT('Ctrl Pts',(58.6189035487885,-11.2205697730928,83.7566656829568));
#3855=CARTESIAN_POINT('Ctrl Pts',(58.6189035487885,-10.7490988661751,84.7087882826478));
#3856=CARTESIAN_POINT('Ctrl Pts',(58.6189035487886,-10.2785552052383,85.1995718651691));
#3857=CARTESIAN_POINT('Ctrl Pts',(58.6189035487886,-9.79907655130654,85.515168675407));
#3858=CARTESIAN_POINT('Ctrl Pts',(58.6189035487886,-9.25227637569268,85.7813082197614));
#3859=CARTESIAN_POINT('Ctrl Pts',(58.6189035487885,-8.12030223033118,86.1208267107997));
#3860=CARTESIAN_POINT('Ctrl Pts',(58.6189035487885,-6.84231551976094,86.2169175365435));
#3861=CARTESIAN_POINT('Ctrl Pts',(58.6189035487885,-5.84860974497664,86.2015080108523));
#3862=CARTESIAN_POINT('Ctrl Pts',(58.6189035487885,-17.1070624647046,75.2236074971792));
#3863=CARTESIAN_POINT('Ctrl Pts',(58.6189035487885,-17.0713749764698,75.2283406973118));
#3864=CARTESIAN_POINT('Ctrl Pts',(58.6189035487885,-17.0356873793413,75.2330738853036));
#3865=CARTESIAN_POINT('Ctrl Pts',(58.6189035487885,-16.868940610655,75.2551744844083));
#3866=CARTESIAN_POINT('Ctrl Pts',(58.6189035487886,-16.6072943602623,75.2878910531892));
#3867=CARTESIAN_POINT('Ctrl Pts',(58.6189035487885,-16.0863108570333,75.3474872987329));
#3868=CARTESIAN_POINT('Ctrl Pts',(58.6189035487885,-15.4407089605501,75.4198407374667));
#3869=CARTESIAN_POINT('Ctrl Pts',(58.6189035487886,-14.810515552782,75.530562741844));
#3870=CARTESIAN_POINT('Ctrl Pts',(58.6189035487885,-14.3226785985763,75.6740330751718));
#3871=CARTESIAN_POINT('Ctrl Pts',(58.6189035487886,-13.6119901077366,75.9531021796814));
#3872=CARTESIAN_POINT('Ctrl Pts',(58.6189035487885,-12.6391386971879,76.6898853504872));
#3873=CARTESIAN_POINT('Ctrl Pts',(58.6189035487886,-11.9421053181931,77.9551448661809));
#3874=CARTESIAN_POINT('Ctrl Pts',(58.6189035487886,-11.620123611833,78.904610366011));
#3875=CARTESIAN_POINT('Ctrl Pts',(58.6189035487886,-11.4414090651326,79.5566822517067));
#3876=CARTESIAN_POINT('Ctrl Pts',(58.6189035487886,-11.283611680672,80.3904836204666));
#3877=CARTESIAN_POINT('Ctrl Pts',(58.6189035487885,-11.191771906312,81.2094324300899));
#3878=CARTESIAN_POINT('Ctrl Pts',(58.6189035487885,-11.1351578812696,81.8374901150816));
#3879=CARTESIAN_POINT('Ctrl Pts',(58.6189035487885,-11.053369822089,82.7460850644104));
#3880=CARTESIAN_POINT('Ctrl Pts',(58.6189035487885,-10.9236831233095,83.6860531538696));
#3881=CARTESIAN_POINT('Ctrl Pts',(58.6189035487885,-10.4992473440377,84.5353425071605));
#3882=CARTESIAN_POINT('Ctrl Pts',(58.6189035487886,-10.0852341421502,84.9682405076987));
#3883=CARTESIAN_POINT('Ctrl Pts',(58.6189035487886,-9.65205447547462,85.2538515396933));
#3884=CARTESIAN_POINT('Ctrl Pts',(58.6189035487886,-9.1488264052405,85.4990822689984));
#3885=CARTESIAN_POINT('Ctrl Pts',(58.6189035487885,-8.07907491053992,85.8217946659718));
#3886=CARTESIAN_POINT('Ctrl Pts',(58.6189035487885,-6.83128625461351,85.9175112317093));
#3887=CARTESIAN_POINT('Ctrl Pts',(58.6189035487885,-5.85324890998301,85.9023446784181));
#3888=CARTESIAN_POINT('Ctrl Pts',(56.7143685644419,-17.0504395293355,74.7966806225093));
#3889=CARTESIAN_POINT('Ctrl Pts',(56.7149839995477,-17.0502694819401,74.795398495354));
#3890=CARTESIAN_POINT('Ctrl Pts',(56.7156024450586,-17.0500996228054,74.7941177876506));
#3891=CARTESIAN_POINT('Ctrl Pts',(56.7162239011616,-17.0499299537481,74.7928385130966));
#3892=CARTESIAN_POINT('Ctrl Pts',(56.8455023604483,-17.0146345334931,74.5267173139489));
#3893=CARTESIAN_POINT('Ctrl Pts',(57.1050624944829,-16.9875646029503,74.3226148461249));
#3894=CARTESIAN_POINT('Ctrl Pts',(57.396117357852,-16.9788276685414,74.2567399126353));
#3895=CARTESIAN_POINT('Ctrl Pts',(57.6696862862663,-16.970615629903,74.1948226000178));
#3896=CARTESIAN_POINT('Ctrl Pts',(57.9710793513523,-16.9785999454106,74.2550229206802));
#3897=CARTESIAN_POINT('Ctrl Pts',(58.1997282611953,-16.9998571535647,74.4152984942149));
#3898=CARTESIAN_POINT('Origin',(57.6189035487885,-17.,75.237807097577));
#3899=CARTESIAN_POINT('',(58.6189035487885,-5.85324890998301,85.9023446784181));
#3900=CARTESIAN_POINT('Ctrl Pts',(58.6189035487885,-17.0000000161406,75.2378038846518));
#3901=CARTESIAN_POINT('Ctrl Pts',(58.6189035487885,-16.868940610655,75.2551744844083));
#3902=CARTESIAN_POINT('Ctrl Pts',(58.6189035487886,-16.6072943602623,75.2878910531892));
#3903=CARTESIAN_POINT('Ctrl Pts',(58.6189035487885,-16.0863108570333,75.3474872987329));
#3904=CARTESIAN_POINT('Ctrl Pts',(58.6189035487885,-15.4407089605501,75.4198407374667));
#3905=CARTESIAN_POINT('Ctrl Pts',(58.6189035487886,-14.810515552782,75.530562741844));
#3906=CARTESIAN_POINT('Ctrl Pts',(58.6189035487885,-14.3226785985763,75.6740330751718));
#3907=CARTESIAN_POINT('Ctrl Pts',(58.6189035487886,-13.6119901077366,75.9531021796814));
#3908=CARTESIAN_POINT('Ctrl Pts',(58.6189035487885,-12.6391386971879,76.6898853504872));
#3909=CARTESIAN_POINT('Ctrl Pts',(58.6189035487886,-11.9421053181931,77.9551448661809));
#3910=CARTESIAN_POINT('Ctrl Pts',(58.6189035487886,-11.620123611833,78.904610366011));
#3911=CARTESIAN_POINT('Ctrl Pts',(58.6189035487886,-11.4414090651326,79.5566822517067));
#3912=CARTESIAN_POINT('Ctrl Pts',(58.6189035487886,-11.283611680672,80.3904836204666));
#3913=CARTESIAN_POINT('Ctrl Pts',(58.6189035487885,-11.191771906312,81.2094324300899));
#3914=CARTESIAN_POINT('Ctrl Pts',(58.6189035487885,-11.1351578812696,81.8374901150816));
#3915=CARTESIAN_POINT('Ctrl Pts',(58.6189035487885,-11.053369822089,82.7460850644104));
#3916=CARTESIAN_POINT('Ctrl Pts',(58.6189035487885,-10.9236831233095,83.6860531538696));
#3917=CARTESIAN_POINT('Ctrl Pts',(58.6189035487885,-10.4992473440377,84.5353425071605));
#3918=CARTESIAN_POINT('Ctrl Pts',(58.6189035487886,-10.0852341421502,84.9682405076987));
#3919=CARTESIAN_POINT('Ctrl Pts',(58.6189035487886,-9.65205447547462,85.2538515396933));
#3920=CARTESIAN_POINT('Ctrl Pts',(58.6189035487886,-9.1488264052405,85.4990822689984));
#3921=CARTESIAN_POINT('Ctrl Pts',(58.6189035487885,-8.07907491053992,85.8217946659718));
#3922=CARTESIAN_POINT('Ctrl Pts',(58.6189035487885,-6.83128625461351,85.9175112317093));
#3923=CARTESIAN_POINT('Ctrl Pts',(58.6189035487885,-5.85324890998301,85.9023446784181));
#3924=CARTESIAN_POINT('Origin',(57.6189035487885,-5.85324890998301,85.9023446784181));
#3925=CARTESIAN_POINT('Ctrl Pts',(57.0348213440502,-17.1658500115857,49.3940081933445));
#3926=CARTESIAN_POINT('Ctrl Pts',(57.036896662294,-17.1105926457513,49.4039659001254));
#3927=CARTESIAN_POINT('Ctrl Pts',(57.0379346870417,-17.0552963237907,49.4139236069063));
#3928=CARTESIAN_POINT('Ctrl Pts',(57.0379346870417,-17.,49.4238813136872));
#3929=CARTESIAN_POINT('Ctrl Pts',(56.8725534287442,-17.1597556645255,49.509914425448));
#3930=CARTESIAN_POINT('Ctrl Pts',(56.874552252259,-17.1065350452187,49.5198721322289));
#3931=CARTESIAN_POINT('Ctrl Pts',(56.8755523684112,-17.0532581413011,49.5298298390098));
#3932=CARTESIAN_POINT('Ctrl Pts',(56.8755523684112,-17.,49.5397875457908));
#3933=CARTESIAN_POINT('Ctrl Pts',(56.6199907504015,-17.1502700886903,49.8416628129442));
#3934=CARTESIAN_POINT('Ctrl Pts',(56.6218712933677,-17.100198803981,49.8516205197251));
#3935=CARTESIAN_POINT('Ctrl Pts',(56.6228116264629,-17.0501065863364,49.861578226506));
#3936=CARTESIAN_POINT('Ctrl Pts',(56.6228116264629,-17.,49.8715359332869));
#3937=CARTESIAN_POINT('Ctrl Pts',(56.5976270641714,-17.1494301687025,50.2581169344504));
#3938=CARTESIAN_POINT('Ctrl Pts',(56.5994965856415,-17.0996523420419,50.2680746412313));
#3939=CARTESIAN_POINT('Ctrl Pts',(56.6004321732215,-17.0498129213918,50.2780323480122));
#3940=CARTESIAN_POINT('Ctrl Pts',(56.6004321732215,-17.,50.2879900547931));
#3941=CARTESIAN_POINT('Ctrl Pts',(56.6462070845395,-17.1512547037855,50.4516083418488));
#3942=CARTESIAN_POINT('Ctrl Pts',(56.6480997684365,-17.1008601549921,50.4615660486297));
#3943=CARTESIAN_POINT('Ctrl Pts',(56.6490464438345,-17.0504300783306,50.4715237554107));
#3944=CARTESIAN_POINT('Ctrl Pts',(56.6490464438345,-17.,50.4814814621916));
#3945=CARTESIAN_POINT('Origin',(57.6189035487885,-17.,50.237807097577));
#3946=CARTESIAN_POINT('Origin',(57.6189035487885,-17.,50.237807097577));
#3947=CARTESIAN_POINT('Origin',(57.6189035487885,-21.7910956063159,41.2894961290256));
#3948=CARTESIAN_POINT('Origin',(57.6189035487885,-17.1070624647042,75.2236074971793));
#3949=CARTESIAN_POINT('',(57.6189035487885,-17.,74.4163755309633));
#3950=CARTESIAN_POINT('Origin',(57.6189035487885,-17.,75.237807097577));
#3951=CARTESIAN_POINT('Origin',(57.6189035487885,-5.85324890998301,85.9023446784181));
#3952=CARTESIAN_POINT('Origin',(57.6189035487885,-17.,75.237807097577));
#4063=UNCERTAINTY_MEASURE_WITH_UNIT(LENGTH_MEASURE(0.01),#4080,
'DISTANCE_ACCURACY_VALUE',
'Maximum model space distance between geometric entities at asserted c
onnectivities');
#4069=UNCERTAINTY_MEASURE_WITH_UNIT(LENGTH_MEASURE(0.01),#4080,
'DISTANCE_ACCURACY_VALUE',
'Maximum model space distance between geometric entities at asserted c
onnectivities');
#4073=(
GEOMETRIC_REPRESENTATION_CONTEXT(3)
GLOBAL_UNCERTAINTY_ASSIGNED_CONTEXT((#4063))
GLOBAL_UNIT_ASSIGNED_CONTEXT((#4080,#4082,#4083))
REPRESENTATION_CONTEXT('','3D')
);
#4079=(
GEOMETRIC_REPRESENTATION_CONTEXT(3)
GLOBAL_UNCERTAINTY_ASSIGNED_CONTEXT((#4069))
GLOBAL_UNIT_ASSIGNED_CONTEXT((#4080,#4082,#4083))
REPRESENTATION_CONTEXT('','3D')
);
#4080=(
LENGTH_UNIT()
NAMED_UNIT(*)
SI_UNIT(.MILLI.,.METRE.)
);
#4082=(
NAMED_UNIT(*)
PLANE_ANGLE_UNIT()
SI_UNIT($,.RADIAN.)
);
#4083=(
NAMED_UNIT(*)
SI_UNIT($,.STERADIAN.)
SOLID_ANGLE_UNIT()
);
#4087=SHAPE_DEFINITION_REPRESENTATION(#4096,#4113);
#4096=PRODUCT_DEFINITION_SHAPE('',$,#4123);
#4113=SHAPE_REPRESENTATION('',(#1632),#4073);
#4119=PRODUCT_DEFINITION_CONTEXT('part definition',#4148,'design');
#4123=PRODUCT_DEFINITION('Spring','Spring',#4132,#4119);
#4132=PRODUCT_DEFINITION_FORMATION('',$,#4153);
#4148=APPLICATION_CONTEXT(
'Core Data for Automotive Mechanical Design Process');
#4149=PRODUCT_CONTEXT('part definition',#4148,'mechanical');
#4153=PRODUCT('Spring','Spring',$,(#4149));
#4162=PRESENTATION_STYLE_ASSIGNMENT((#4166));
#4166=SURFACE_STYLE_USAGE(.BOTH.,#4170);
#4170=SURFACE_SIDE_STYLE('',(#4174));
#4174=SURFACE_STYLE_FILL_AREA(#4178);
#4178=FILL_AREA_STYLE('Stainless Steel - Satin',(#4182));
#4182=FILL_AREA_STYLE_COLOUR('Stainless Steel - Satin',#4186);
#4186=COLOUR_RGB('Stainless Steel - Satin', 0.31764706, 0.68627451, 0.89019608);
ENDSEC;
END-ISO-10303-21;
